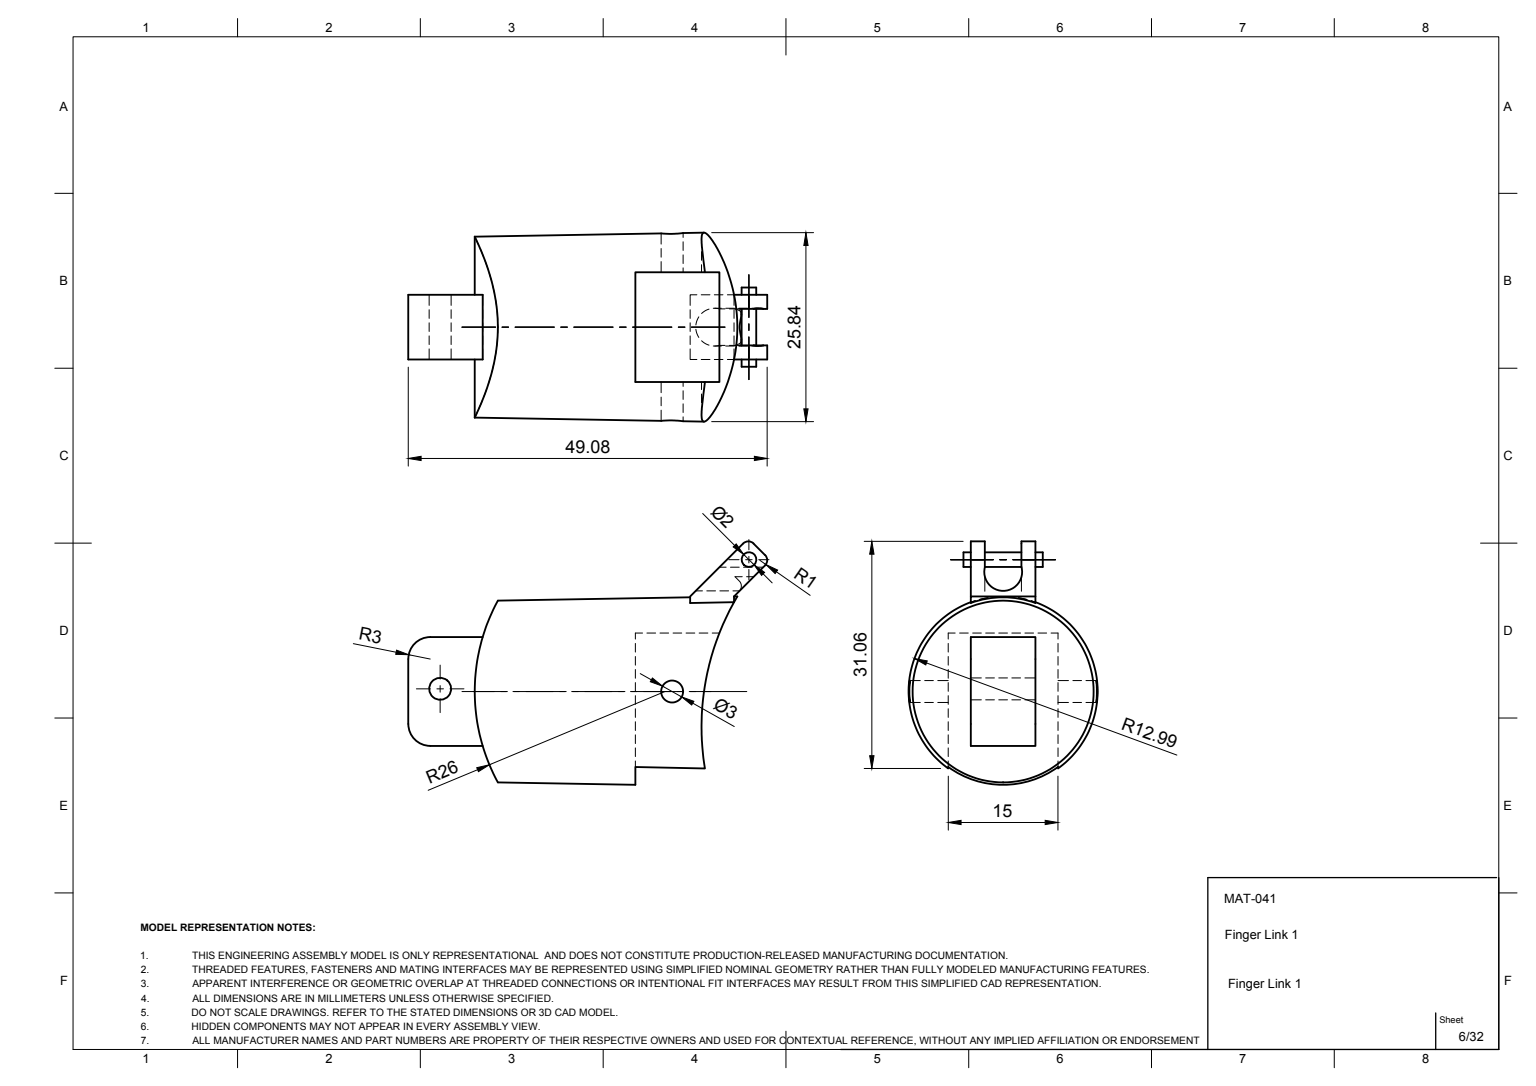
ISO-10303-21;
HEADER;
/* Generated by software containing ST-Developer
 * from STEP Tools, Inc. (www.steptools.com) 
 */

FILE_DESCRIPTION(
/* description */ ('STEP AP214'),
/* implementation_level */ '2;1');

FILE_NAME(
/* name */ 'Finger Link 1.step',
/* time_stamp */ '2026-11-14T21:57:47-08:00',
/* author */ (''),
/* organization */ (''),
/* preprocessor_version */ 'ST-DEVELOPER v20.2',
/* originating_system */ 'Autodesk Translation Framework v15.17.0.0',
/* authorisation */ '');

FILE_SCHEMA (('AUTOMOTIVE_DESIGN { 1 0 10303 214 3 1 1 }'));
ENDSEC;

DATA;
#10=MECHANICAL_DESIGN_GEOMETRIC_PRESENTATION_REPRESENTATION('',(#249),#13199);
#117=CONICAL_SURFACE('',#7216,13.,0.0174532925199433);
#118=CONICAL_SURFACE('',#7226,13.,0.0174532925199433);
#127=B_SPLINE_CURVE_WITH_KNOTS('',3,(#10160,#10161,#10162,#10163,#10164,
#10165,#10166,#10167,#10168,#10169,#10170,#10171,#10172,#10173,#10174,#10175,
#10176,#10177),.UNSPECIFIED.,.F.,.F.,(4,2,2,2,2,2,2,2,4),(-0.625948273254299,
-0.595286193065165,-0.532168206431192,-0.441842646589546,-0.3515170867479,
-0.261191526906255,-0.170865967064609,-0.107747980430636,-0.0770859002412175),
 .UNSPECIFIED.);
#128=B_SPLINE_CURVE_WITH_KNOTS('',3,(#10225,#10226,#10227,#10228,#10229,
#10230,#10231,#10232,#10233,#10234,#10235,#10236,#10237,#10238,#10239,#10240,
#10241,#10242),.UNSPECIFIED.,.F.,.F.,(4,2,2,2,2,2,2,2,4),(1.130849455016,
1.18732607982086,1.24380270462571,1.30024878607951,1.35669486753331,1.41336679321831,
1.4700387189033,1.52669509758432,1.58335147626535),.UNSPECIFIED.);
#129=B_SPLINE_CURVE_WITH_KNOTS('',3,(#10243,#10244,#10245,#10246,#10247,
#10248,#10249,#10250,#10251,#10252,#10253,#10254,#10255,#10256,#10257,#10258,
#10259,#10260,#10261),.UNSPECIFIED.,.F.,.F.,(4,2,2,2,3,2,2,2,4),(0.678347433766657,
0.735003812447681,0.791660191128705,0.848332116813698,0.905004042498691,
0.961450123952495,1.0178962054063,1.07437283021115,1.130849455016),
 .UNSPECIFIED.);
#130=B_SPLINE_CURVE_WITH_KNOTS('',3,(#10265,#10266,#10267,#10268,#10269,
#10270,#10271,#10272,#10273,#10274,#10275,#10276,#10277,#10278,#10279,#10280,
#10281,#10282),.UNSPECIFIED.,.F.,.F.,(4,2,2,2,2,2,2,2,4),(-0.678347433766657,
-0.621691055085633,-0.565034676404609,-0.508362750719616,-0.451690825034623,
-0.39524474358082,-0.338798662127016,-0.282322037322164,-0.225845412517312),
 .UNSPECIFIED.);
#131=B_SPLINE_CURVE_WITH_KNOTS('',3,(#10286,#10287,#10288,#10289,#10290,
#10291,#10292,#10293,#10294,#10295,#10296,#10297,#10298,#10299,#10300,#10301,
#10302,#10303,#10304),.UNSPECIFIED.,.F.,.F.,(4,2,2,2,3,2,2,2,4),(-0.225845412517312,
-0.169368787712459,-0.112892162907607,-0.0564460814538034,0.,0.0566719256849931,
0.113343851369986,0.17000023005101,0.226656608732034),.UNSPECIFIED.);
#132=B_SPLINE_CURVE_WITH_KNOTS('',3,(#10310,#10311,#10312,#10313),
 .UNSPECIFIED.,.F.,.F.,(4,4),(0.0270217399274549,0.0365389400069035),
 .UNSPECIFIED.);
#133=B_SPLINE_CURVE_WITH_KNOTS('',3,(#10315,#10316,#10317,#10318,#10319,
#10320,#10321,#10322,#10323,#10324,#10325,#10326,#10327,#10328,#10329,#10330,
#10331,#10332),.UNSPECIFIED.,.F.,.F.,(4,2,2,2,2,2,2,2,4),(4.40493642535816,
4.46219553041876,4.95875793037621,5.46800962865692,5.97726132693763,6.22066748237464,
6.46407363781164,6.95088594868566,7.16462957817159),.UNSPECIFIED.);
#134=B_SPLINE_CURVE_WITH_KNOTS('',3,(#10334,#10335,#10336,#10337,#10338,
#10339,#10340),.UNSPECIFIED.,.F.,.F.,(4,3,4),(0.0223867113798144,0.0254340142714909,
0.0283877461116507),.UNSPECIFIED.);
#135=B_SPLINE_CURVE_WITH_KNOTS('',3,(#10346,#10347,#10348,#10349,#10350,
#10351,#10352,#10353,#10354,#10355,#10356,#10357,#10358,#10359,#10360,#10361,
#10362,#10363,#10364,#10365,#10366,#10367,#10368,#10369,#10370,#10371),
 .UNSPECIFIED.,.F.,.F.,(4,2,2,2,2,2,2,2,2,2,2,2,4),(3.80610647446318,4.04439914990187,
4.28269182534056,4.75927717621793,5.2342149273987,5.47168380298909,5.70915267857947,
5.94662421983221,6.18409576108494,6.65903884359041,7.13562589625839,7.37391942259238,
7.61221294892637),.UNSPECIFIED.);
#136=B_SPLINE_CURVE_WITH_KNOTS('',3,(#10372,#10373,#10374,#10375,#10376,
#10377,#10378,#10379,#10380,#10381,#10382,#10383,#10384,#10385,#10386,#10387,
#10388,#10389,#10390,#10391,#10392,#10393,#10394,#10395,#10396,#10397),
 .UNSPECIFIED.,.F.,.F.,(4,2,2,2,2,2,2,2,2,2,2,2,4),(0.,0.238293526333989,
0.476587052667979,0.953174105335958,1.42811718784143,1.66558872909416,1.90306027034689,
2.14052914593728,2.37799802152767,2.85293577270844,3.32952112358581,3.5678137990245,
3.80610647446318),.UNSPECIFIED.);
#137=B_SPLINE_CURVE_WITH_KNOTS('',3,(#10401,#10402,#10403,#10404,#10405,
#10406,#10407),.UNSPECIFIED.,.F.,.F.,(4,3,4),(0.0224802824352469,0.0254340142749992,
0.0284813171662554),.UNSPECIFIED.);
#138=B_SPLINE_CURVE_WITH_KNOTS('',3,(#10409,#10410,#10411,#10412,#10413,
#10414,#10415,#10416,#10417,#10418,#10419,#10420,#10421,#10422,#10423,#10424,
#10425,#10426),.UNSPECIFIED.,.F.,.F.,(4,2,2,2,2,2,2,2,4),(0.766636682751041,
0.98038031223697,1.46719262311099,1.710598778548,1.95400493398501,2.46325663226571,
2.97250833054642,3.46907073050387,3.52632983556447),.UNSPECIFIED.);
#139=B_SPLINE_CURVE_WITH_KNOTS('',3,(#10427,#10428,#10429,#10430),
 .UNSPECIFIED.,.F.,.F.,(4,4),(0.0143722070064857,0.0238894070520057),
 .UNSPECIFIED.);
#140=B_SPLINE_CURVE_WITH_KNOTS('',3,(#10456,#10457,#10458,#10459,#10460,
#10461,#10462,#10463,#10464,#10465),.UNSPECIFIED.,.F.,.F.,(4,2,2,2,4),(3.52632983556447,
3.71735193048259,3.96563313046132,4.21391433044004,4.40493642535816),
 .UNSPECIFIED.);
#213=SHAPE_REPRESENTATION_RELATIONSHIP('SRR','None',#13281,#231);
#231=ADVANCED_BREP_SHAPE_REPRESENTATION('',(#267),#13177);
#249=STYLED_ITEM('',(#13409),#267);
#267=MANIFOLD_SOLID_BREP('Body1',#6844);
#290=FACE_BOUND('',#2265,.T.);
#291=FACE_BOUND('',#2266,.T.);
#292=FACE_BOUND('',#2274,.T.);
#293=FACE_BOUND('',#2277,.T.);
#294=FACE_BOUND('',#2279,.T.);
#295=FACE_BOUND('',#2283,.T.);
#296=FACE_BOUND('',#2286,.T.);
#297=FACE_BOUND('',#2292,.T.);
#298=FACE_BOUND('',#2294,.T.);
#299=FACE_BOUND('',#2304,.T.);
#300=FACE_BOUND('',#2307,.T.);
#387=ELLIPSE('',#7195,3.65324790347504,2.58323636587766);
#388=ELLIPSE('',#7196,3.65324790353112,2.58323636594297);
#389=ELLIPSE('',#7197,3.65324790353033,2.58323636594184);
#390=ELLIPSE('',#7198,3.65324790353218,2.58323636594453);
#391=ELLIPSE('',#7199,3.65324790349574,2.58323636589973);
#416=PLANE('',#7220);
#417=PLANE('',#7221);
#418=PLANE('',#7223);
#419=PLANE('',#7225);
#420=PLANE('',#7234);
#421=PLANE('',#7235);
#422=PLANE('',#7236);
#423=PLANE('',#7237);
#424=PLANE('',#7238);
#425=PLANE('',#7239);
#426=PLANE('',#7242);
#427=PLANE('',#7243);
#428=PLANE('',#7246);
#429=PLANE('',#7247);
#430=PLANE('',#7248);
#431=PLANE('',#7249);
#432=PLANE('',#7250);
#433=PLANE('',#7253);
#434=PLANE('',#7256);
#435=PLANE('',#7257);
#436=PLANE('',#7263);
#437=PLANE('',#7264);
#438=PLANE('',#7267);
#439=PLANE('',#7268);
#440=PLANE('',#7271);
#672=LINE('',#10181,#1190);
#673=LINE('',#10185,#1191);
#674=LINE('',#10189,#1192);
#675=LINE('',#10193,#1193);
#676=LINE('',#10199,#1194);
#677=LINE('',#10205,#1195);
#678=LINE('',#10211,#1196);
#679=LINE('',#10217,#1197);
#680=LINE('',#10223,#1198);
#681=LINE('',#10284,#1199);
#682=LINE('',#10344,#1200);
#683=LINE('',#10433,#1201);
#684=LINE('',#10434,#1202);
#685=LINE('',#10437,#1203);
#686=LINE('',#10441,#1204);
#687=LINE('',#10443,#1205);
#688=LINE('',#10448,#1206);
#689=LINE('',#10450,#1207);
#690=LINE('',#10452,#1208);
#691=LINE('',#10453,#1209);
#692=LINE('',#10469,#1210);
#693=LINE('',#10475,#1211);
#694=LINE('',#10479,#1212);
#695=LINE('',#10483,#1213);
#696=LINE('',#10485,#1214);
#697=LINE('',#10486,#1215);
#698=LINE('',#10488,#1216);
#699=LINE('',#10490,#1217);
#700=LINE('',#10494,#1218);
#701=LINE('',#10496,#1219);
#702=LINE('',#10497,#1220);
#703=LINE('',#10501,#1221);
#704=LINE('',#10505,#1222);
#705=LINE('',#10506,#1223);
#706=LINE('',#10508,#1224);
#707=LINE('',#10512,#1225);
#708=LINE('',#10513,#1226);
#709=LINE('',#10516,#1227);
#710=LINE('',#10520,#1228);
#711=LINE('',#10523,#1229);
#712=LINE('',#10524,#1230);
#713=LINE('',#10526,#1231);
#714=LINE('',#10527,#1232);
#715=LINE('',#10528,#1233);
#716=LINE('',#10531,#1234);
#717=LINE('',#10533,#1235);
#718=LINE('',#10534,#1236);
#719=LINE('',#10535,#1237);
#720=LINE('',#10539,#1238);
#721=LINE('',#10540,#1239);
#722=LINE('',#10541,#1240);
#723=LINE('',#10543,#1241);
#724=LINE('',#10560,#1242);
#725=LINE('',#10562,#1243);
#726=LINE('',#10564,#1244);
#727=LINE('',#10565,#1245);
#728=LINE('',#10568,#1246);
#729=LINE('',#10572,#1247);
#730=LINE('',#10575,#1248);
#731=LINE('',#10576,#1249);
#732=LINE('',#10580,#1250);
#733=LINE('',#10583,#1251);
#1190=VECTOR('',#8163,1000.);
#1191=VECTOR('',#8166,1000.);
#1192=VECTOR('',#8169,1000.);
#1193=VECTOR('',#8172,1000.);
#1194=VECTOR('',#8179,1.5);
#1195=VECTOR('',#8186,1.);
#1196=VECTOR('',#8193,1.);
#1197=VECTOR('',#8200,1.);
#1198=VECTOR('',#8207,1.5);
#1199=VECTOR('',#8210,1.5);
#1200=VECTOR('',#8219,13.);
#1201=VECTOR('',#8224,1000.);
#1202=VECTOR('',#8225,1000.);
#1203=VECTOR('',#8228,1000.);
#1204=VECTOR('',#8233,1000.);
#1205=VECTOR('',#8234,1000.);
#1206=VECTOR('',#8239,1000.);
#1207=VECTOR('',#8240,1000.);
#1208=VECTOR('',#8241,1000.);
#1209=VECTOR('',#8242,1000.);
#1210=VECTOR('',#8249,1000.);
#1211=VECTOR('',#8256,1000.);
#1212=VECTOR('',#8259,1000.);
#1213=VECTOR('',#8264,1000.);
#1214=VECTOR('',#8265,1000.);
#1215=VECTOR('',#8266,1000.);
#1216=VECTOR('',#8269,1000.);
#1217=VECTOR('',#8272,1000.);
#1218=VECTOR('',#8277,1000.);
#1219=VECTOR('',#8278,1000.);
#1220=VECTOR('',#8279,1000.);
#1221=VECTOR('',#8282,1000.);
#1222=VECTOR('',#8285,1000.);
#1223=VECTOR('',#8286,1000.);
#1224=VECTOR('',#8287,1000.);
#1225=VECTOR('',#8292,1000.);
#1226=VECTOR('',#8293,1000.);
#1227=VECTOR('',#8296,1000.);
#1228=VECTOR('',#8301,1000.);
#1229=VECTOR('',#8304,1000.);
#1230=VECTOR('',#8305,1000.);
#1231=VECTOR('',#8306,1000.);
#1232=VECTOR('',#8307,1000.);
#1233=VECTOR('',#8308,1000.);
#1234=VECTOR('',#8311,1000.);
#1235=VECTOR('',#8312,1000.);
#1236=VECTOR('',#8313,1000.);
#1237=VECTOR('',#8314,1000.);
#1238=VECTOR('',#8317,1000.);
#1239=VECTOR('',#8318,1000.);
#1240=VECTOR('',#8319,1000.);
#1241=VECTOR('',#8322,1000.);
#1242=VECTOR('',#8351,1000.);
#1243=VECTOR('',#8352,1000.);
#1244=VECTOR('',#8353,1000.);
#1245=VECTOR('',#8354,1000.);
#1246=VECTOR('',#8357,1000.);
#1247=VECTOR('',#8362,1000.);
#1248=VECTOR('',#8365,1000.);
#1249=VECTOR('',#8366,1000.);
#1250=VECTOR('',#8371,1000.);
#1251=VECTOR('',#8376,1000.);
#1669=CYLINDRICAL_SURFACE('',#7194,2.58323636594183);
#1670=CYLINDRICAL_SURFACE('',#7200,1.5);
#1671=CYLINDRICAL_SURFACE('',#7203,1.);
#1672=CYLINDRICAL_SURFACE('',#7206,1.);
#1673=CYLINDRICAL_SURFACE('',#7209,1.);
#1674=CYLINDRICAL_SURFACE('',#7212,1.5);
#1675=CYLINDRICAL_SURFACE('',#7214,1.5);
#1676=CYLINDRICAL_SURFACE('',#7228,35.);
#1677=CYLINDRICAL_SURFACE('',#7231,26.);
#1678=CYLINDRICAL_SURFACE('',#7258,1.);
#1679=CYLINDRICAL_SURFACE('',#7259,1.);
#1680=CYLINDRICAL_SURFACE('',#7260,1.);
#1681=CYLINDRICAL_SURFACE('',#7261,1.);
#1682=CYLINDRICAL_SURFACE('',#7262,1.);
#1683=CYLINDRICAL_SURFACE('',#7272,3.);
#1684=CYLINDRICAL_SURFACE('',#7273,3.);
#1860=FACE_OUTER_BOUND('',#2257,.T.);
#1861=FACE_OUTER_BOUND('',#2258,.T.);
#1862=FACE_OUTER_BOUND('',#2259,.T.);
#1863=FACE_OUTER_BOUND('',#2260,.T.);
#1864=FACE_OUTER_BOUND('',#2261,.T.);
#1865=FACE_OUTER_BOUND('',#2262,.T.);
#1866=FACE_OUTER_BOUND('',#2263,.T.);
#1867=FACE_OUTER_BOUND('',#2264,.T.);
#1868=FACE_OUTER_BOUND('',#2267,.T.);
#1869=FACE_OUTER_BOUND('',#2268,.T.);
#1870=FACE_OUTER_BOUND('',#2269,.T.);
#1871=FACE_OUTER_BOUND('',#2270,.T.);
#1872=FACE_OUTER_BOUND('',#2271,.T.);
#1873=FACE_OUTER_BOUND('',#2272,.T.);
#1874=FACE_OUTER_BOUND('',#2273,.T.);
#1875=FACE_OUTER_BOUND('',#2275,.T.);
#1876=FACE_OUTER_BOUND('',#2276,.T.);
#1877=FACE_OUTER_BOUND('',#2278,.T.);
#1878=FACE_OUTER_BOUND('',#2280,.T.);
#1879=FACE_OUTER_BOUND('',#2281,.T.);
#1880=FACE_OUTER_BOUND('',#2282,.T.);
#1881=FACE_OUTER_BOUND('',#2284,.T.);
#1882=FACE_OUTER_BOUND('',#2285,.T.);
#1883=FACE_OUTER_BOUND('',#2287,.T.);
#1884=FACE_OUTER_BOUND('',#2288,.T.);
#1885=FACE_OUTER_BOUND('',#2289,.T.);
#1886=FACE_OUTER_BOUND('',#2290,.T.);
#1887=FACE_OUTER_BOUND('',#2291,.T.);
#1888=FACE_OUTER_BOUND('',#2293,.T.);
#1889=FACE_OUTER_BOUND('',#2295,.T.);
#1890=FACE_OUTER_BOUND('',#2296,.T.);
#1891=FACE_OUTER_BOUND('',#2297,.T.);
#1892=FACE_OUTER_BOUND('',#2298,.T.);
#1893=FACE_OUTER_BOUND('',#2299,.T.);
#1894=FACE_OUTER_BOUND('',#2300,.T.);
#1895=FACE_OUTER_BOUND('',#2301,.T.);
#1896=FACE_OUTER_BOUND('',#2302,.T.);
#1897=FACE_OUTER_BOUND('',#2303,.T.);
#1898=FACE_OUTER_BOUND('',#2305,.T.);
#1899=FACE_OUTER_BOUND('',#2306,.T.);
#1900=FACE_OUTER_BOUND('',#2308,.T.);
#1901=FACE_OUTER_BOUND('',#2309,.T.);
#1902=FACE_OUTER_BOUND('',#2310,.T.);
#2257=EDGE_LOOP('',(#4822,#4823,#4824,#4825,#4826,#4827,#4828,#4829,#4830,
#4831));
#2258=EDGE_LOOP('',(#4832,#4833,#4834,#4835));
#2259=EDGE_LOOP('',(#4836,#4837,#4838,#4839));
#2260=EDGE_LOOP('',(#4840,#4841,#4842,#4843));
#2261=EDGE_LOOP('',(#4844,#4845,#4846,#4847));
#2262=EDGE_LOOP('',(#4848,#4849,#4850,#4851,#4852));
#2263=EDGE_LOOP('',(#4853,#4854,#4855,#4856,#4857));
#2264=EDGE_LOOP('',(#4858,#4859,#4860,#4861,#4862,#4863,#4864,#4865,#4866,
#4867,#4868,#4869,#4870));
#2265=EDGE_LOOP('',(#4871,#4872));
#2266=EDGE_LOOP('',(#4873,#4874));
#2267=EDGE_LOOP('',(#4875,#4876,#4877));
#2268=EDGE_LOOP('',(#4878,#4879,#4880,#4881));
#2269=EDGE_LOOP('',(#4882,#4883,#4884,#4885));
#2270=EDGE_LOOP('',(#4886,#4887,#4888,#4889));
#2271=EDGE_LOOP('',(#4890,#4891));
#2272=EDGE_LOOP('',(#4892,#4893,#4894,#4895,#4896,#4897));
#2273=EDGE_LOOP('',(#4898,#4899));
#2274=EDGE_LOOP('',(#4900,#4901,#4902,#4903));
#2275=EDGE_LOOP('',(#4904,#4905,#4906,#4907));
#2276=EDGE_LOOP('',(#4908,#4909,#4910,#4911));
#2277=EDGE_LOOP('',(#4912));
#2278=EDGE_LOOP('',(#4913,#4914,#4915,#4916));
#2279=EDGE_LOOP('',(#4917));
#2280=EDGE_LOOP('',(#4918,#4919,#4920,#4921));
#2281=EDGE_LOOP('',(#4922,#4923,#4924,#4925));
#2282=EDGE_LOOP('',(#4926,#4927,#4928,#4929,#4930,#4931,#4932,#4933));
#2283=EDGE_LOOP('',(#4934));
#2284=EDGE_LOOP('',(#4935,#4936,#4937,#4938,#4939));
#2285=EDGE_LOOP('',(#4940,#4941,#4942,#4943,#4944,#4945,#4946,#4947));
#2286=EDGE_LOOP('',(#4948));
#2287=EDGE_LOOP('',(#4949,#4950,#4951,#4952,#4953,#4954,#4955,#4956,#4957,
#4958,#4959,#4960));
#2288=EDGE_LOOP('',(#4961,#4962,#4963,#4964,#4965,#4966,#4967,#4968));
#2289=EDGE_LOOP('',(#4969,#4970,#4971,#4972));
#2290=EDGE_LOOP('',(#4973,#4974,#4975));
#2291=EDGE_LOOP('',(#4976,#4977,#4978,#4979,#4980,#4981));
#2292=EDGE_LOOP('',(#4982));
#2293=EDGE_LOOP('',(#4983,#4984,#4985,#4986,#4987,#4988));
#2294=EDGE_LOOP('',(#4989));
#2295=EDGE_LOOP('',(#4990));
#2296=EDGE_LOOP('',(#4991));
#2297=EDGE_LOOP('',(#4992,#4993,#4994,#4995));
#2298=EDGE_LOOP('',(#4996,#4997,#4998,#4999));
#2299=EDGE_LOOP('',(#5000,#5001,#5002,#5003));
#2300=EDGE_LOOP('',(#5004,#5005,#5006,#5007));
#2301=EDGE_LOOP('',(#5008,#5009,#5010,#5011,#5012,#5013));
#2302=EDGE_LOOP('',(#5014,#5015,#5016,#5017));
#2303=EDGE_LOOP('',(#5018,#5019,#5020,#5021,#5022,#5023));
#2304=EDGE_LOOP('',(#5024));
#2305=EDGE_LOOP('',(#5025,#5026,#5027,#5028));
#2306=EDGE_LOOP('',(#5029,#5030,#5031,#5032,#5033,#5034));
#2307=EDGE_LOOP('',(#5035));
#2308=EDGE_LOOP('',(#5036,#5037,#5038,#5039));
#2309=EDGE_LOOP('',(#5040,#5041,#5042,#5043));
#2310=EDGE_LOOP('',(#5044,#5045,#5046,#5047));
#2747=CIRCLE('',#7201,1.5);
#2748=CIRCLE('',#7202,1.5);
#2749=CIRCLE('',#7204,1.);
#2750=CIRCLE('',#7205,1.);
#2751=CIRCLE('',#7207,1.);
#2752=CIRCLE('',#7208,1.);
#2753=CIRCLE('',#7210,1.);
#2754=CIRCLE('',#7211,1.);
#2755=CIRCLE('',#7213,1.5);
#2756=CIRCLE('',#7215,1.5);
#2757=CIRCLE('',#7217,12.7565008166693);
#2758=CIRCLE('',#7218,12.8874008156035);
#2759=CIRCLE('',#7219,12.8874008156035);
#2760=CIRCLE('',#7222,1.);
#2761=CIRCLE('',#7224,1.);
#2762=CIRCLE('',#7227,12.9921312051728);
#2763=CIRCLE('',#7229,35.);
#2764=CIRCLE('',#7230,35.);
#2765=CIRCLE('',#7232,26.);
#2766=CIRCLE('',#7233,26.);
#2767=CIRCLE('',#7240,1.);
#2768=CIRCLE('',#7241,1.);
#2769=CIRCLE('',#7244,1.);
#2770=CIRCLE('',#7245,1.);
#2771=CIRCLE('',#7251,1.);
#2772=CIRCLE('',#7252,1.);
#2773=CIRCLE('',#7254,1.);
#2774=CIRCLE('',#7255,1.);
#2775=CIRCLE('',#7265,3.);
#2776=CIRCLE('',#7266,3.);
#2777=CIRCLE('',#7269,3.);
#2778=CIRCLE('',#7270,3.);
#3076=VERTEX_POINT('',#10158);
#3077=VERTEX_POINT('',#10159);
#3078=VERTEX_POINT('',#10178);
#3079=VERTEX_POINT('',#10180);
#3080=VERTEX_POINT('',#10182);
#3081=VERTEX_POINT('',#10184);
#3082=VERTEX_POINT('',#10186);
#3083=VERTEX_POINT('',#10188);
#3084=VERTEX_POINT('',#10190);
#3085=VERTEX_POINT('',#10192);
#3086=VERTEX_POINT('',#10196);
#3087=VERTEX_POINT('',#10198);
#3088=VERTEX_POINT('',#10202);
#3089=VERTEX_POINT('',#10204);
#3090=VERTEX_POINT('',#10208);
#3091=VERTEX_POINT('',#10210);
#3092=VERTEX_POINT('',#10214);
#3093=VERTEX_POINT('',#10216);
#3094=VERTEX_POINT('',#10220);
#3095=VERTEX_POINT('',#10222);
#3096=VERTEX_POINT('',#10224);
#3097=VERTEX_POINT('',#10263);
#3098=VERTEX_POINT('',#10264);
#3099=VERTEX_POINT('',#10283);
#3100=VERTEX_POINT('',#10306);
#3101=VERTEX_POINT('',#10307);
#3102=VERTEX_POINT('',#10309);
#3103=VERTEX_POINT('',#10314);
#3104=VERTEX_POINT('',#10333);
#3105=VERTEX_POINT('',#10341);
#3106=VERTEX_POINT('',#10343);
#3107=VERTEX_POINT('',#10345);
#3108=VERTEX_POINT('',#10398);
#3109=VERTEX_POINT('',#10400);
#3110=VERTEX_POINT('',#10408);
#3111=VERTEX_POINT('',#10432);
#3112=VERTEX_POINT('',#10436);
#3113=VERTEX_POINT('',#10440);
#3114=VERTEX_POINT('',#10442);
#3115=VERTEX_POINT('',#10446);
#3116=VERTEX_POINT('',#10447);
#3117=VERTEX_POINT('',#10449);
#3118=VERTEX_POINT('',#10451);
#3119=VERTEX_POINT('',#10467);
#3120=VERTEX_POINT('',#10468);
#3121=VERTEX_POINT('',#10473);
#3122=VERTEX_POINT('',#10474);
#3123=VERTEX_POINT('',#10476);
#3124=VERTEX_POINT('',#10478);
#3125=VERTEX_POINT('',#10482);
#3126=VERTEX_POINT('',#10484);
#3127=VERTEX_POINT('',#10493);
#3128=VERTEX_POINT('',#10495);
#3129=VERTEX_POINT('',#10499);
#3130=VERTEX_POINT('',#10500);
#3131=VERTEX_POINT('',#10502);
#3132=VERTEX_POINT('',#10504);
#3133=VERTEX_POINT('',#10507);
#3134=VERTEX_POINT('',#10511);
#3135=VERTEX_POINT('',#10515);
#3136=VERTEX_POINT('',#10518);
#3137=VERTEX_POINT('',#10522);
#3138=VERTEX_POINT('',#10525);
#3139=VERTEX_POINT('',#10530);
#3140=VERTEX_POINT('',#10532);
#3141=VERTEX_POINT('',#10537);
#3142=VERTEX_POINT('',#10538);
#3143=VERTEX_POINT('',#10558);
#3144=VERTEX_POINT('',#10559);
#3145=VERTEX_POINT('',#10561);
#3146=VERTEX_POINT('',#10563);
#3147=VERTEX_POINT('',#10567);
#3148=VERTEX_POINT('',#10570);
#3149=VERTEX_POINT('',#10574);
#3150=VERTEX_POINT('',#10579);
#3748=EDGE_CURVE('',#3076,#3077,#127,.T.);
#3749=EDGE_CURVE('',#3078,#3077,#387,.T.);
#3750=EDGE_CURVE('',#3079,#3078,#672,.T.);
#3751=EDGE_CURVE('',#3080,#3079,#388,.T.);
#3752=EDGE_CURVE('',#3080,#3081,#673,.T.);
#3753=EDGE_CURVE('',#3082,#3081,#389,.T.);
#3754=EDGE_CURVE('',#3083,#3082,#674,.T.);
#3755=EDGE_CURVE('',#3084,#3083,#390,.T.);
#3756=EDGE_CURVE('',#3085,#3084,#675,.T.);
#3757=EDGE_CURVE('',#3076,#3085,#391,.T.);
#3758=EDGE_CURVE('',#3086,#3086,#2747,.T.);
#3759=EDGE_CURVE('',#3086,#3087,#676,.T.);
#3760=EDGE_CURVE('',#3087,#3087,#2748,.T.);
#3761=EDGE_CURVE('',#3088,#3088,#2749,.T.);
#3762=EDGE_CURVE('',#3088,#3089,#677,.T.);
#3763=EDGE_CURVE('',#3089,#3089,#2750,.T.);
#3764=EDGE_CURVE('',#3090,#3090,#2751,.T.);
#3765=EDGE_CURVE('',#3090,#3091,#678,.T.);
#3766=EDGE_CURVE('',#3091,#3091,#2752,.T.);
#3767=EDGE_CURVE('',#3092,#3092,#2753,.T.);
#3768=EDGE_CURVE('',#3092,#3093,#679,.T.);
#3769=EDGE_CURVE('',#3093,#3093,#2754,.T.);
#3770=EDGE_CURVE('',#3094,#3094,#2755,.T.);
#3771=EDGE_CURVE('',#3094,#3095,#680,.T.);
#3772=EDGE_CURVE('',#3095,#3096,#128,.T.);
#3773=EDGE_CURVE('',#3096,#3095,#129,.T.);
#3774=EDGE_CURVE('',#3097,#3098,#130,.T.);
#3775=EDGE_CURVE('',#3098,#3099,#681,.T.);
#3776=EDGE_CURVE('',#3099,#3099,#2756,.T.);
#3777=EDGE_CURVE('',#3098,#3097,#131,.T.);
#3778=EDGE_CURVE('',#3100,#3101,#2757,.T.);
#3779=EDGE_CURVE('',#3102,#3100,#132,.T.);
#3780=EDGE_CURVE('',#3103,#3102,#133,.T.);
#3781=EDGE_CURVE('',#3103,#3104,#134,.T.);
#3782=EDGE_CURVE('',#3104,#3105,#2758,.T.);
#3783=EDGE_CURVE('',#3105,#3106,#682,.T.);
#3784=EDGE_CURVE('',#3106,#3107,#135,.T.);
#3785=EDGE_CURVE('',#3107,#3106,#136,.T.);
#3786=EDGE_CURVE('',#3105,#3108,#2759,.T.);
#3787=EDGE_CURVE('',#3108,#3109,#137,.T.);
#3788=EDGE_CURVE('',#3110,#3109,#138,.T.);
#3789=EDGE_CURVE('',#3101,#3110,#139,.T.);
#3790=EDGE_CURVE('',#3111,#3078,#683,.T.);
#3791=EDGE_CURVE('',#3077,#3111,#684,.T.);
#3792=EDGE_CURVE('',#3079,#3112,#685,.T.);
#3793=EDGE_CURVE('',#3111,#3112,#2760,.T.);
#3794=EDGE_CURVE('',#3113,#3085,#686,.T.);
#3795=EDGE_CURVE('',#3114,#3084,#687,.T.);
#3796=EDGE_CURVE('',#3114,#3113,#2761,.T.);
#3797=EDGE_CURVE('',#3115,#3116,#688,.T.);
#3798=EDGE_CURVE('',#3116,#3117,#689,.T.);
#3799=EDGE_CURVE('',#3118,#3117,#690,.T.);
#3800=EDGE_CURVE('',#3118,#3115,#691,.T.);
#3801=EDGE_CURVE('',#3109,#3103,#2762,.T.);
#3802=EDGE_CURVE('',#3109,#3103,#140,.T.);
#3803=EDGE_CURVE('',#3119,#3120,#692,.T.);
#3804=EDGE_CURVE('',#3119,#3110,#2763,.T.);
#3805=EDGE_CURVE('',#3102,#3120,#2764,.T.);
#3806=EDGE_CURVE('',#3121,#3122,#693,.T.);
#3807=EDGE_CURVE('',#3123,#3121,#2765,.T.);
#3808=EDGE_CURVE('',#3124,#3123,#694,.T.);
#3809=EDGE_CURVE('',#3122,#3124,#2766,.T.);
#3810=EDGE_CURVE('',#3101,#3125,#695,.T.);
#3811=EDGE_CURVE('',#3126,#3125,#696,.T.);
#3812=EDGE_CURVE('',#3100,#3126,#697,.T.);
#3813=EDGE_CURVE('',#3125,#3119,#698,.T.);
#3814=EDGE_CURVE('',#3120,#3126,#699,.T.);
#3815=EDGE_CURVE('',#3109,#3127,#700,.T.);
#3816=EDGE_CURVE('',#3127,#3128,#701,.T.);
#3817=EDGE_CURVE('',#3103,#3128,#702,.T.);
#3818=EDGE_CURVE('',#3129,#3130,#703,.T.);
#3819=EDGE_CURVE('',#3129,#3131,#2767,.T.);
#3820=EDGE_CURVE('',#3131,#3132,#704,.T.);
#3821=EDGE_CURVE('',#3104,#3132,#705,.T.);
#3822=EDGE_CURVE('',#3133,#3128,#706,.T.);
#3823=EDGE_CURVE('',#3133,#3130,#2768,.T.);
#3824=EDGE_CURVE('',#3132,#3134,#707,.T.);
#3825=EDGE_CURVE('',#3108,#3134,#708,.T.);
#3826=EDGE_CURVE('',#3135,#3134,#709,.T.);
#3827=EDGE_CURVE('',#3135,#3116,#2769,.T.);
#3828=EDGE_CURVE('',#3115,#3136,#2770,.T.);
#3829=EDGE_CURVE('',#3136,#3127,#710,.T.);
#3830=EDGE_CURVE('',#3083,#3137,#711,.T.);
#3831=EDGE_CURVE('',#3137,#3133,#712,.T.);
#3832=EDGE_CURVE('',#3136,#3138,#713,.T.);
#3833=EDGE_CURVE('',#3138,#3080,#714,.T.);
#3834=EDGE_CURVE('',#3112,#3114,#715,.T.);
#3835=EDGE_CURVE('',#3082,#3139,#716,.T.);
#3836=EDGE_CURVE('',#3140,#3081,#717,.T.);
#3837=EDGE_CURVE('',#3140,#3135,#718,.T.);
#3838=EDGE_CURVE('',#3131,#3139,#719,.T.);
#3839=EDGE_CURVE('',#3141,#3142,#720,.T.);
#3840=EDGE_CURVE('',#3141,#3129,#721,.T.);
#3841=EDGE_CURVE('',#3130,#3142,#722,.T.);
#3842=EDGE_CURVE('',#3113,#3076,#723,.T.);
#3843=EDGE_CURVE('',#3138,#3118,#2771,.T.);
#3844=EDGE_CURVE('',#3117,#3140,#2772,.T.);
#3845=EDGE_CURVE('',#3139,#3141,#2773,.T.);
#3846=EDGE_CURVE('',#3142,#3137,#2774,.T.);
#3847=EDGE_CURVE('',#3143,#3144,#724,.T.);
#3848=EDGE_CURVE('',#3144,#3145,#725,.T.);
#3849=EDGE_CURVE('',#3145,#3146,#726,.T.);
#3850=EDGE_CURVE('',#3146,#3143,#727,.T.);
#3851=EDGE_CURVE('',#3121,#3147,#728,.T.);
#3852=EDGE_CURVE('',#3147,#3144,#2775,.T.);
#3853=EDGE_CURVE('',#3143,#3148,#2776,.T.);
#3854=EDGE_CURVE('',#3123,#3148,#729,.T.);
#3855=EDGE_CURVE('',#3122,#3149,#730,.T.);
#3856=EDGE_CURVE('',#3149,#3147,#731,.T.);
#3857=EDGE_CURVE('',#3145,#3149,#2777,.T.);
#3858=EDGE_CURVE('',#3124,#3150,#732,.T.);
#3859=EDGE_CURVE('',#3150,#3146,#2778,.T.);
#3860=EDGE_CURVE('',#3148,#3150,#733,.T.);
#4822=ORIENTED_EDGE('',*,*,#3748,.T.);
#4823=ORIENTED_EDGE('',*,*,#3749,.F.);
#4824=ORIENTED_EDGE('',*,*,#3750,.F.);
#4825=ORIENTED_EDGE('',*,*,#3751,.F.);
#4826=ORIENTED_EDGE('',*,*,#3752,.T.);
#4827=ORIENTED_EDGE('',*,*,#3753,.F.);
#4828=ORIENTED_EDGE('',*,*,#3754,.F.);
#4829=ORIENTED_EDGE('',*,*,#3755,.F.);
#4830=ORIENTED_EDGE('',*,*,#3756,.F.);
#4831=ORIENTED_EDGE('',*,*,#3757,.F.);
#4832=ORIENTED_EDGE('',*,*,#3758,.T.);
#4833=ORIENTED_EDGE('',*,*,#3759,.T.);
#4834=ORIENTED_EDGE('',*,*,#3760,.T.);
#4835=ORIENTED_EDGE('',*,*,#3759,.F.);
#4836=ORIENTED_EDGE('',*,*,#3761,.T.);
#4837=ORIENTED_EDGE('',*,*,#3762,.T.);
#4838=ORIENTED_EDGE('',*,*,#3763,.T.);
#4839=ORIENTED_EDGE('',*,*,#3762,.F.);
#4840=ORIENTED_EDGE('',*,*,#3764,.T.);
#4841=ORIENTED_EDGE('',*,*,#3765,.T.);
#4842=ORIENTED_EDGE('',*,*,#3766,.F.);
#4843=ORIENTED_EDGE('',*,*,#3765,.F.);
#4844=ORIENTED_EDGE('',*,*,#3767,.T.);
#4845=ORIENTED_EDGE('',*,*,#3768,.T.);
#4846=ORIENTED_EDGE('',*,*,#3769,.T.);
#4847=ORIENTED_EDGE('',*,*,#3768,.F.);
#4848=ORIENTED_EDGE('',*,*,#3770,.F.);
#4849=ORIENTED_EDGE('',*,*,#3771,.T.);
#4850=ORIENTED_EDGE('',*,*,#3772,.T.);
#4851=ORIENTED_EDGE('',*,*,#3773,.T.);
#4852=ORIENTED_EDGE('',*,*,#3771,.F.);
#4853=ORIENTED_EDGE('',*,*,#3774,.T.);
#4854=ORIENTED_EDGE('',*,*,#3775,.T.);
#4855=ORIENTED_EDGE('',*,*,#3776,.F.);
#4856=ORIENTED_EDGE('',*,*,#3775,.F.);
#4857=ORIENTED_EDGE('',*,*,#3777,.T.);
#4858=ORIENTED_EDGE('',*,*,#3778,.F.);
#4859=ORIENTED_EDGE('',*,*,#3779,.F.);
#4860=ORIENTED_EDGE('',*,*,#3780,.F.);
#4861=ORIENTED_EDGE('',*,*,#3781,.T.);
#4862=ORIENTED_EDGE('',*,*,#3782,.T.);
#4863=ORIENTED_EDGE('',*,*,#3783,.T.);
#4864=ORIENTED_EDGE('',*,*,#3784,.T.);
#4865=ORIENTED_EDGE('',*,*,#3785,.T.);
#4866=ORIENTED_EDGE('',*,*,#3783,.F.);
#4867=ORIENTED_EDGE('',*,*,#3786,.T.);
#4868=ORIENTED_EDGE('',*,*,#3787,.T.);
#4869=ORIENTED_EDGE('',*,*,#3788,.F.);
#4870=ORIENTED_EDGE('',*,*,#3789,.F.);
#4871=ORIENTED_EDGE('',*,*,#3774,.F.);
#4872=ORIENTED_EDGE('',*,*,#3777,.F.);
#4873=ORIENTED_EDGE('',*,*,#3773,.F.);
#4874=ORIENTED_EDGE('',*,*,#3772,.F.);
#4875=ORIENTED_EDGE('',*,*,#3790,.T.);
#4876=ORIENTED_EDGE('',*,*,#3749,.T.);
#4877=ORIENTED_EDGE('',*,*,#3791,.T.);
#4878=ORIENTED_EDGE('',*,*,#3792,.F.);
#4879=ORIENTED_EDGE('',*,*,#3750,.T.);
#4880=ORIENTED_EDGE('',*,*,#3790,.F.);
#4881=ORIENTED_EDGE('',*,*,#3793,.T.);
#4882=ORIENTED_EDGE('',*,*,#3794,.T.);
#4883=ORIENTED_EDGE('',*,*,#3756,.T.);
#4884=ORIENTED_EDGE('',*,*,#3795,.F.);
#4885=ORIENTED_EDGE('',*,*,#3796,.T.);
#4886=ORIENTED_EDGE('',*,*,#3797,.T.);
#4887=ORIENTED_EDGE('',*,*,#3798,.T.);
#4888=ORIENTED_EDGE('',*,*,#3799,.F.);
#4889=ORIENTED_EDGE('',*,*,#3800,.T.);
#4890=ORIENTED_EDGE('',*,*,#3801,.T.);
#4891=ORIENTED_EDGE('',*,*,#3802,.F.);
#4892=ORIENTED_EDGE('',*,*,#3803,.F.);
#4893=ORIENTED_EDGE('',*,*,#3804,.T.);
#4894=ORIENTED_EDGE('',*,*,#3788,.T.);
#4895=ORIENTED_EDGE('',*,*,#3802,.T.);
#4896=ORIENTED_EDGE('',*,*,#3780,.T.);
#4897=ORIENTED_EDGE('',*,*,#3805,.T.);
#4898=ORIENTED_EDGE('',*,*,#3785,.F.);
#4899=ORIENTED_EDGE('',*,*,#3784,.F.);
#4900=ORIENTED_EDGE('',*,*,#3806,.F.);
#4901=ORIENTED_EDGE('',*,*,#3807,.F.);
#4902=ORIENTED_EDGE('',*,*,#3808,.F.);
#4903=ORIENTED_EDGE('',*,*,#3809,.F.);
#4904=ORIENTED_EDGE('',*,*,#3778,.T.);
#4905=ORIENTED_EDGE('',*,*,#3810,.T.);
#4906=ORIENTED_EDGE('',*,*,#3811,.F.);
#4907=ORIENTED_EDGE('',*,*,#3812,.F.);
#4908=ORIENTED_EDGE('',*,*,#3789,.T.);
#4909=ORIENTED_EDGE('',*,*,#3804,.F.);
#4910=ORIENTED_EDGE('',*,*,#3813,.F.);
#4911=ORIENTED_EDGE('',*,*,#3810,.F.);
#4912=ORIENTED_EDGE('',*,*,#3770,.T.);
#4913=ORIENTED_EDGE('',*,*,#3779,.T.);
#4914=ORIENTED_EDGE('',*,*,#3812,.T.);
#4915=ORIENTED_EDGE('',*,*,#3814,.F.);
#4916=ORIENTED_EDGE('',*,*,#3805,.F.);
#4917=ORIENTED_EDGE('',*,*,#3776,.T.);
#4918=ORIENTED_EDGE('',*,*,#3803,.T.);
#4919=ORIENTED_EDGE('',*,*,#3814,.T.);
#4920=ORIENTED_EDGE('',*,*,#3811,.T.);
#4921=ORIENTED_EDGE('',*,*,#3813,.T.);
#4922=ORIENTED_EDGE('',*,*,#3801,.F.);
#4923=ORIENTED_EDGE('',*,*,#3815,.T.);
#4924=ORIENTED_EDGE('',*,*,#3816,.T.);
#4925=ORIENTED_EDGE('',*,*,#3817,.F.);
#4926=ORIENTED_EDGE('',*,*,#3818,.F.);
#4927=ORIENTED_EDGE('',*,*,#3819,.T.);
#4928=ORIENTED_EDGE('',*,*,#3820,.T.);
#4929=ORIENTED_EDGE('',*,*,#3821,.F.);
#4930=ORIENTED_EDGE('',*,*,#3781,.F.);
#4931=ORIENTED_EDGE('',*,*,#3817,.T.);
#4932=ORIENTED_EDGE('',*,*,#3822,.F.);
#4933=ORIENTED_EDGE('',*,*,#3823,.T.);
#4934=ORIENTED_EDGE('',*,*,#3763,.F.);
#4935=ORIENTED_EDGE('',*,*,#3782,.F.);
#4936=ORIENTED_EDGE('',*,*,#3821,.T.);
#4937=ORIENTED_EDGE('',*,*,#3824,.T.);
#4938=ORIENTED_EDGE('',*,*,#3825,.F.);
#4939=ORIENTED_EDGE('',*,*,#3786,.F.);
#4940=ORIENTED_EDGE('',*,*,#3826,.F.);
#4941=ORIENTED_EDGE('',*,*,#3827,.T.);
#4942=ORIENTED_EDGE('',*,*,#3797,.F.);
#4943=ORIENTED_EDGE('',*,*,#3828,.T.);
#4944=ORIENTED_EDGE('',*,*,#3829,.T.);
#4945=ORIENTED_EDGE('',*,*,#3815,.F.);
#4946=ORIENTED_EDGE('',*,*,#3787,.F.);
#4947=ORIENTED_EDGE('',*,*,#3825,.T.);
#4948=ORIENTED_EDGE('',*,*,#3764,.F.);
#4949=ORIENTED_EDGE('',*,*,#3795,.T.);
#4950=ORIENTED_EDGE('',*,*,#3755,.T.);
#4951=ORIENTED_EDGE('',*,*,#3830,.T.);
#4952=ORIENTED_EDGE('',*,*,#3831,.T.);
#4953=ORIENTED_EDGE('',*,*,#3822,.T.);
#4954=ORIENTED_EDGE('',*,*,#3816,.F.);
#4955=ORIENTED_EDGE('',*,*,#3829,.F.);
#4956=ORIENTED_EDGE('',*,*,#3832,.T.);
#4957=ORIENTED_EDGE('',*,*,#3833,.T.);
#4958=ORIENTED_EDGE('',*,*,#3751,.T.);
#4959=ORIENTED_EDGE('',*,*,#3792,.T.);
#4960=ORIENTED_EDGE('',*,*,#3834,.T.);
#4961=ORIENTED_EDGE('',*,*,#3835,.F.);
#4962=ORIENTED_EDGE('',*,*,#3753,.T.);
#4963=ORIENTED_EDGE('',*,*,#3836,.F.);
#4964=ORIENTED_EDGE('',*,*,#3837,.T.);
#4965=ORIENTED_EDGE('',*,*,#3826,.T.);
#4966=ORIENTED_EDGE('',*,*,#3824,.F.);
#4967=ORIENTED_EDGE('',*,*,#3820,.F.);
#4968=ORIENTED_EDGE('',*,*,#3838,.T.);
#4969=ORIENTED_EDGE('',*,*,#3839,.F.);
#4970=ORIENTED_EDGE('',*,*,#3840,.T.);
#4971=ORIENTED_EDGE('',*,*,#3818,.T.);
#4972=ORIENTED_EDGE('',*,*,#3841,.T.);
#4973=ORIENTED_EDGE('',*,*,#3842,.T.);
#4974=ORIENTED_EDGE('',*,*,#3757,.T.);
#4975=ORIENTED_EDGE('',*,*,#3794,.F.);
#4976=ORIENTED_EDGE('',*,*,#3836,.T.);
#4977=ORIENTED_EDGE('',*,*,#3752,.F.);
#4978=ORIENTED_EDGE('',*,*,#3833,.F.);
#4979=ORIENTED_EDGE('',*,*,#3843,.T.);
#4980=ORIENTED_EDGE('',*,*,#3799,.T.);
#4981=ORIENTED_EDGE('',*,*,#3844,.T.);
#4982=ORIENTED_EDGE('',*,*,#3769,.F.);
#4983=ORIENTED_EDGE('',*,*,#3830,.F.);
#4984=ORIENTED_EDGE('',*,*,#3754,.T.);
#4985=ORIENTED_EDGE('',*,*,#3835,.T.);
#4986=ORIENTED_EDGE('',*,*,#3845,.T.);
#4987=ORIENTED_EDGE('',*,*,#3839,.T.);
#4988=ORIENTED_EDGE('',*,*,#3846,.T.);
#4989=ORIENTED_EDGE('',*,*,#3767,.F.);
#4990=ORIENTED_EDGE('',*,*,#3766,.T.);
#4991=ORIENTED_EDGE('',*,*,#3761,.F.);
#4992=ORIENTED_EDGE('',*,*,#3845,.F.);
#4993=ORIENTED_EDGE('',*,*,#3838,.F.);
#4994=ORIENTED_EDGE('',*,*,#3819,.F.);
#4995=ORIENTED_EDGE('',*,*,#3840,.F.);
#4996=ORIENTED_EDGE('',*,*,#3827,.F.);
#4997=ORIENTED_EDGE('',*,*,#3837,.F.);
#4998=ORIENTED_EDGE('',*,*,#3844,.F.);
#4999=ORIENTED_EDGE('',*,*,#3798,.F.);
#5000=ORIENTED_EDGE('',*,*,#3843,.F.);
#5001=ORIENTED_EDGE('',*,*,#3832,.F.);
#5002=ORIENTED_EDGE('',*,*,#3828,.F.);
#5003=ORIENTED_EDGE('',*,*,#3800,.F.);
#5004=ORIENTED_EDGE('',*,*,#3823,.F.);
#5005=ORIENTED_EDGE('',*,*,#3831,.F.);
#5006=ORIENTED_EDGE('',*,*,#3846,.F.);
#5007=ORIENTED_EDGE('',*,*,#3841,.F.);
#5008=ORIENTED_EDGE('',*,*,#3748,.F.);
#5009=ORIENTED_EDGE('',*,*,#3842,.F.);
#5010=ORIENTED_EDGE('',*,*,#3796,.F.);
#5011=ORIENTED_EDGE('',*,*,#3834,.F.);
#5012=ORIENTED_EDGE('',*,*,#3793,.F.);
#5013=ORIENTED_EDGE('',*,*,#3791,.F.);
#5014=ORIENTED_EDGE('',*,*,#3847,.T.);
#5015=ORIENTED_EDGE('',*,*,#3848,.T.);
#5016=ORIENTED_EDGE('',*,*,#3849,.T.);
#5017=ORIENTED_EDGE('',*,*,#3850,.T.);
#5018=ORIENTED_EDGE('',*,*,#3851,.T.);
#5019=ORIENTED_EDGE('',*,*,#3852,.T.);
#5020=ORIENTED_EDGE('',*,*,#3847,.F.);
#5021=ORIENTED_EDGE('',*,*,#3853,.T.);
#5022=ORIENTED_EDGE('',*,*,#3854,.F.);
#5023=ORIENTED_EDGE('',*,*,#3807,.T.);
#5024=ORIENTED_EDGE('',*,*,#3760,.F.);
#5025=ORIENTED_EDGE('',*,*,#3855,.T.);
#5026=ORIENTED_EDGE('',*,*,#3856,.T.);
#5027=ORIENTED_EDGE('',*,*,#3851,.F.);
#5028=ORIENTED_EDGE('',*,*,#3806,.T.);
#5029=ORIENTED_EDGE('',*,*,#3849,.F.);
#5030=ORIENTED_EDGE('',*,*,#3857,.T.);
#5031=ORIENTED_EDGE('',*,*,#3855,.F.);
#5032=ORIENTED_EDGE('',*,*,#3809,.T.);
#5033=ORIENTED_EDGE('',*,*,#3858,.T.);
#5034=ORIENTED_EDGE('',*,*,#3859,.T.);
#5035=ORIENTED_EDGE('',*,*,#3758,.F.);
#5036=ORIENTED_EDGE('',*,*,#3854,.T.);
#5037=ORIENTED_EDGE('',*,*,#3860,.T.);
#5038=ORIENTED_EDGE('',*,*,#3858,.F.);
#5039=ORIENTED_EDGE('',*,*,#3808,.T.);
#5040=ORIENTED_EDGE('',*,*,#3852,.F.);
#5041=ORIENTED_EDGE('',*,*,#3856,.F.);
#5042=ORIENTED_EDGE('',*,*,#3857,.F.);
#5043=ORIENTED_EDGE('',*,*,#3848,.F.);
#5044=ORIENTED_EDGE('',*,*,#3859,.F.);
#5045=ORIENTED_EDGE('',*,*,#3860,.F.);
#5046=ORIENTED_EDGE('',*,*,#3853,.F.);
#5047=ORIENTED_EDGE('',*,*,#3850,.F.);
#6512=ADVANCED_FACE('',(#1860),#1669,.F.);
#6513=ADVANCED_FACE('',(#1861),#1670,.F.);
#6514=ADVANCED_FACE('',(#1862),#1671,.T.);
#6515=ADVANCED_FACE('',(#1863),#1672,.T.);
#6516=ADVANCED_FACE('',(#1864),#1673,.T.);
#6517=ADVANCED_FACE('',(#1865),#1674,.F.);
#6518=ADVANCED_FACE('',(#1866),#1675,.F.);
#6519=ADVANCED_FACE('',(#1867,#290,#291),#117,.T.);
#6520=ADVANCED_FACE('',(#1868),#416,.F.);
#6521=ADVANCED_FACE('',(#1869),#417,.F.);
#6522=ADVANCED_FACE('',(#1870),#418,.F.);
#6523=ADVANCED_FACE('',(#1871),#419,.T.);
#6524=ADVANCED_FACE('',(#1872),#118,.T.);
#6525=ADVANCED_FACE('',(#1873),#1676,.F.);
#6526=ADVANCED_FACE('',(#1874,#292),#1677,.T.);
#6527=ADVANCED_FACE('',(#1875),#420,.T.);
#6528=ADVANCED_FACE('',(#1876,#293),#421,.T.);
#6529=ADVANCED_FACE('',(#1877,#294),#422,.T.);
#6530=ADVANCED_FACE('',(#1878),#423,.F.);
#6531=ADVANCED_FACE('',(#1879),#424,.F.);
#6532=ADVANCED_FACE('',(#1880,#295),#425,.F.);
#6533=ADVANCED_FACE('',(#1881),#426,.F.);
#6534=ADVANCED_FACE('',(#1882,#296),#427,.F.);
#6535=ADVANCED_FACE('',(#1883),#428,.F.);
#6536=ADVANCED_FACE('',(#1884),#429,.F.);
#6537=ADVANCED_FACE('',(#1885),#430,.T.);
#6538=ADVANCED_FACE('',(#1886),#431,.F.);
#6539=ADVANCED_FACE('',(#1887,#297),#432,.F.);
#6540=ADVANCED_FACE('',(#1888,#298),#433,.F.);
#6541=ADVANCED_FACE('',(#1889),#434,.T.);
#6542=ADVANCED_FACE('',(#1890),#435,.F.);
#6543=ADVANCED_FACE('',(#1891),#1678,.T.);
#6544=ADVANCED_FACE('',(#1892),#1679,.T.);
#6545=ADVANCED_FACE('',(#1893),#1680,.T.);
#6546=ADVANCED_FACE('',(#1894),#1681,.T.);
#6547=ADVANCED_FACE('',(#1895),#1682,.T.);
#6548=ADVANCED_FACE('',(#1896),#436,.F.);
#6549=ADVANCED_FACE('',(#1897,#299),#437,.T.);
#6550=ADVANCED_FACE('',(#1898),#438,.T.);
#6551=ADVANCED_FACE('',(#1899,#300),#439,.T.);
#6552=ADVANCED_FACE('',(#1900),#440,.T.);
#6553=ADVANCED_FACE('',(#1901),#1683,.T.);
#6554=ADVANCED_FACE('',(#1902),#1684,.T.);
#6844=CLOSED_SHELL('',(#6512,#6513,#6514,#6515,#6516,#6517,#6518,#6519,
#6520,#6521,#6522,#6523,#6524,#6525,#6526,#6527,#6528,#6529,#6530,#6531,
#6532,#6533,#6534,#6535,#6536,#6537,#6538,#6539,#6540,#6541,#6542,#6543,
#6544,#6545,#6546,#6547,#6548,#6549,#6550,#6551,#6552,#6553,#6554));
#7193=AXIS2_PLACEMENT_3D('',#10156,#8157,#8158);
#7194=AXIS2_PLACEMENT_3D('',#10157,#8159,#8160);
#7195=AXIS2_PLACEMENT_3D('',#10179,#8161,#8162);
#7196=AXIS2_PLACEMENT_3D('',#10183,#8164,#8165);
#7197=AXIS2_PLACEMENT_3D('',#10187,#8167,#8168);
#7198=AXIS2_PLACEMENT_3D('',#10191,#8170,#8171);
#7199=AXIS2_PLACEMENT_3D('',#10194,#8173,#8174);
#7200=AXIS2_PLACEMENT_3D('',#10195,#8175,#8176);
#7201=AXIS2_PLACEMENT_3D('',#10197,#8177,#8178);
#7202=AXIS2_PLACEMENT_3D('',#10200,#8180,#8181);
#7203=AXIS2_PLACEMENT_3D('',#10201,#8182,#8183);
#7204=AXIS2_PLACEMENT_3D('',#10203,#8184,#8185);
#7205=AXIS2_PLACEMENT_3D('',#10206,#8187,#8188);
#7206=AXIS2_PLACEMENT_3D('',#10207,#8189,#8190);
#7207=AXIS2_PLACEMENT_3D('',#10209,#8191,#8192);
#7208=AXIS2_PLACEMENT_3D('',#10212,#8194,#8195);
#7209=AXIS2_PLACEMENT_3D('',#10213,#8196,#8197);
#7210=AXIS2_PLACEMENT_3D('',#10215,#8198,#8199);
#7211=AXIS2_PLACEMENT_3D('',#10218,#8201,#8202);
#7212=AXIS2_PLACEMENT_3D('',#10219,#8203,#8204);
#7213=AXIS2_PLACEMENT_3D('',#10221,#8205,#8206);
#7214=AXIS2_PLACEMENT_3D('',#10262,#8208,#8209);
#7215=AXIS2_PLACEMENT_3D('',#10285,#8211,#8212);
#7216=AXIS2_PLACEMENT_3D('',#10305,#8213,#8214);
#7217=AXIS2_PLACEMENT_3D('',#10308,#8215,#8216);
#7218=AXIS2_PLACEMENT_3D('',#10342,#8217,#8218);
#7219=AXIS2_PLACEMENT_3D('',#10399,#8220,#8221);
#7220=AXIS2_PLACEMENT_3D('',#10431,#8222,#8223);
#7221=AXIS2_PLACEMENT_3D('',#10435,#8226,#8227);
#7222=AXIS2_PLACEMENT_3D('',#10438,#8229,#8230);
#7223=AXIS2_PLACEMENT_3D('',#10439,#8231,#8232);
#7224=AXIS2_PLACEMENT_3D('',#10444,#8235,#8236);
#7225=AXIS2_PLACEMENT_3D('',#10445,#8237,#8238);
#7226=AXIS2_PLACEMENT_3D('',#10454,#8243,#8244);
#7227=AXIS2_PLACEMENT_3D('',#10455,#8245,#8246);
#7228=AXIS2_PLACEMENT_3D('',#10466,#8247,#8248);
#7229=AXIS2_PLACEMENT_3D('',#10470,#8250,#8251);
#7230=AXIS2_PLACEMENT_3D('',#10471,#8252,#8253);
#7231=AXIS2_PLACEMENT_3D('',#10472,#8254,#8255);
#7232=AXIS2_PLACEMENT_3D('',#10477,#8257,#8258);
#7233=AXIS2_PLACEMENT_3D('',#10480,#8260,#8261);
#7234=AXIS2_PLACEMENT_3D('',#10481,#8262,#8263);
#7235=AXIS2_PLACEMENT_3D('',#10487,#8267,#8268);
#7236=AXIS2_PLACEMENT_3D('',#10489,#8270,#8271);
#7237=AXIS2_PLACEMENT_3D('',#10491,#8273,#8274);
#7238=AXIS2_PLACEMENT_3D('',#10492,#8275,#8276);
#7239=AXIS2_PLACEMENT_3D('',#10498,#8280,#8281);
#7240=AXIS2_PLACEMENT_3D('',#10503,#8283,#8284);
#7241=AXIS2_PLACEMENT_3D('',#10509,#8288,#8289);
#7242=AXIS2_PLACEMENT_3D('',#10510,#8290,#8291);
#7243=AXIS2_PLACEMENT_3D('',#10514,#8294,#8295);
#7244=AXIS2_PLACEMENT_3D('',#10517,#8297,#8298);
#7245=AXIS2_PLACEMENT_3D('',#10519,#8299,#8300);
#7246=AXIS2_PLACEMENT_3D('',#10521,#8302,#8303);
#7247=AXIS2_PLACEMENT_3D('',#10529,#8309,#8310);
#7248=AXIS2_PLACEMENT_3D('',#10536,#8315,#8316);
#7249=AXIS2_PLACEMENT_3D('',#10542,#8320,#8321);
#7250=AXIS2_PLACEMENT_3D('',#10544,#8323,#8324);
#7251=AXIS2_PLACEMENT_3D('',#10545,#8325,#8326);
#7252=AXIS2_PLACEMENT_3D('',#10546,#8327,#8328);
#7253=AXIS2_PLACEMENT_3D('',#10547,#8329,#8330);
#7254=AXIS2_PLACEMENT_3D('',#10548,#8331,#8332);
#7255=AXIS2_PLACEMENT_3D('',#10549,#8333,#8334);
#7256=AXIS2_PLACEMENT_3D('',#10550,#8335,#8336);
#7257=AXIS2_PLACEMENT_3D('',#10551,#8337,#8338);
#7258=AXIS2_PLACEMENT_3D('',#10552,#8339,#8340);
#7259=AXIS2_PLACEMENT_3D('',#10553,#8341,#8342);
#7260=AXIS2_PLACEMENT_3D('',#10554,#8343,#8344);
#7261=AXIS2_PLACEMENT_3D('',#10555,#8345,#8346);
#7262=AXIS2_PLACEMENT_3D('',#10556,#8347,#8348);
#7263=AXIS2_PLACEMENT_3D('',#10557,#8349,#8350);
#7264=AXIS2_PLACEMENT_3D('',#10566,#8355,#8356);
#7265=AXIS2_PLACEMENT_3D('',#10569,#8358,#8359);
#7266=AXIS2_PLACEMENT_3D('',#10571,#8360,#8361);
#7267=AXIS2_PLACEMENT_3D('',#10573,#8363,#8364);
#7268=AXIS2_PLACEMENT_3D('',#10577,#8367,#8368);
#7269=AXIS2_PLACEMENT_3D('',#10578,#8369,#8370);
#7270=AXIS2_PLACEMENT_3D('',#10581,#8372,#8373);
#7271=AXIS2_PLACEMENT_3D('',#10582,#8374,#8375);
#7272=AXIS2_PLACEMENT_3D('',#10584,#8377,#8378);
#7273=AXIS2_PLACEMENT_3D('',#10585,#8379,#8380);
#8157=DIRECTION('axis',(0.,0.,1.));
#8158=DIRECTION('refdir',(1.,0.,0.));
#8159=DIRECTION('center_axis',(0.,0.,1.));
#8160=DIRECTION('ref_axis',(1.,0.,0.));
#8161=DIRECTION('center_axis',(0.707106781186558,-5.01171544695272E-14,
0.707106781186537));
#8162=DIRECTION('ref_axis',(0.707106781186537,1.30563837326012E-11,-0.707106781186558));
#8163=DIRECTION('',(0.,0.,1.));
#8164=DIRECTION('center_axis',(-0.707106781186548,-3.66800410274155E-14,
0.707106781186547));
#8165=DIRECTION('ref_axis',(0.707106781186547,-1.32695584283249E-13,0.707106781186548));
#8166=DIRECTION('',(0.,0.,1.));
#8167=DIRECTION('center_axis',(0.707106781186548,-2.49447284670762E-16,
-0.707106781186547));
#8168=DIRECTION('ref_axis',(0.707106781186547,3.43199962798826E-15,0.707106781186548));
#8169=DIRECTION('',(0.,0.,1.));
#8170=DIRECTION('center_axis',(-0.707106781186548,-5.83546107254331E-15,
0.707106781186547));
#8171=DIRECTION('ref_axis',(0.707106781186547,-8.39541658988548E-14,0.707106781186548));
#8172=DIRECTION('',(0.,0.,-1.));
#8173=DIRECTION('center_axis',(0.70710678118654,-3.75878658521447E-14,0.707106781186555));
#8174=DIRECTION('ref_axis',(0.707106781186555,-7.50458522379288E-12,-0.70710678118654));
#8175=DIRECTION('center_axis',(0.,-1.,0.));
#8176=DIRECTION('ref_axis',(0.,0.,-1.));
#8177=DIRECTION('center_axis',(0.,1.,0.));
#8178=DIRECTION('ref_axis',(0.,0.,1.));
#8179=DIRECTION('',(0.,-1.,0.));
#8180=DIRECTION('center_axis',(0.,-1.,0.));
#8181=DIRECTION('ref_axis',(0.,0.,-1.));
#8182=DIRECTION('center_axis',(0.,1.,0.));
#8183=DIRECTION('ref_axis',(0.,0.,1.));
#8184=DIRECTION('center_axis',(0.,-1.,0.));
#8185=DIRECTION('ref_axis',(0.,0.,-1.));
#8186=DIRECTION('',(0.,-1.,0.));
#8187=DIRECTION('center_axis',(0.,1.,0.));
#8188=DIRECTION('ref_axis',(0.,0.,-1.));
#8189=DIRECTION('center_axis',(0.,1.,0.));
#8190=DIRECTION('ref_axis',(0.,0.,1.));
#8191=DIRECTION('center_axis',(0.,-1.,0.));
#8192=DIRECTION('ref_axis',(0.,0.,1.));
#8193=DIRECTION('',(0.,-1.,0.));
#8194=DIRECTION('center_axis',(0.,-1.,0.));
#8195=DIRECTION('ref_axis',(0.,0.,-1.));
#8196=DIRECTION('center_axis',(0.,1.,0.));
#8197=DIRECTION('ref_axis',(0.,0.,1.));
#8198=DIRECTION('center_axis',(0.,-1.,0.));
#8199=DIRECTION('ref_axis',(0.,0.,1.));
#8200=DIRECTION('',(0.,-1.,0.));
#8201=DIRECTION('center_axis',(0.,1.,0.));
#8202=DIRECTION('ref_axis',(0.,0.,-1.));
#8203=DIRECTION('center_axis',(0.,-1.,0.));
#8204=DIRECTION('ref_axis',(0.,0.,-1.));
#8205=DIRECTION('center_axis',(0.,-1.,-1.24352412568707E-16));
#8206=DIRECTION('ref_axis',(0.,-1.24352412568707E-16,1.));
#8207=DIRECTION('',(0.,-1.,0.));
#8208=DIRECTION('center_axis',(0.,-1.,0.));
#8209=DIRECTION('ref_axis',(0.,0.,-1.));
#8210=DIRECTION('',(0.,-1.,0.));
#8211=DIRECTION('center_axis',(0.,1.,1.24352412568707E-16));
#8212=DIRECTION('ref_axis',(0.,1.24352412568707E-16,-1.));
#8213=DIRECTION('center_axis',(0.,0.,-1.));
#8214=DIRECTION('ref_axis',(1.,0.,0.));
#8215=DIRECTION('center_axis',(0.,1.15648231731787E-16,-1.));
#8216=DIRECTION('ref_axis',(0.,1.,1.15648231731787E-16));
#8217=DIRECTION('center_axis',(0.,0.,1.));
#8218=DIRECTION('ref_axis',(-1.,0.,0.));
#8219=DIRECTION('',(0.0174524064372835,-2.1373033680838E-18,0.999847695156391));
#8220=DIRECTION('center_axis',(0.,0.,1.));
#8221=DIRECTION('ref_axis',(-1.,0.,0.));
#8222=DIRECTION('center_axis',(0.707106781186548,0.,0.707106781186548));
#8223=DIRECTION('ref_axis',(0.707106781186548,0.,-0.707106781186548));
#8224=DIRECTION('',(-0.707106781186547,0.,0.707106781186547));
#8225=DIRECTION('',(0.,-1.,0.));
#8226=DIRECTION('center_axis',(0.,-1.,0.));
#8227=DIRECTION('ref_axis',(0.,0.,-1.));
#8228=DIRECTION('',(0.707106781186548,0.,0.707106781186548));
#8229=DIRECTION('center_axis',(0.,-1.,0.));
#8230=DIRECTION('ref_axis',(0.,0.,-1.));
#8231=DIRECTION('center_axis',(0.,1.,0.));
#8232=DIRECTION('ref_axis',(0.,0.,1.));
#8233=DIRECTION('',(-0.707106781186547,0.,0.707106781186547));
#8234=DIRECTION('',(-0.707106781186548,0.,-0.707106781186548));
#8235=DIRECTION('center_axis',(0.,1.,0.));
#8236=DIRECTION('ref_axis',(0.,0.,1.));
#8237=DIRECTION('center_axis',(-0.707106781186547,0.,-0.707106781186548));
#8238=DIRECTION('ref_axis',(-0.707106781186548,0.,0.707106781186547));
#8239=DIRECTION('',(-0.707106781186548,0.,0.707106781186547));
#8240=DIRECTION('',(0.,1.,0.));
#8241=DIRECTION('',(-0.707106781186548,0.,0.707106781186547));
#8242=DIRECTION('',(0.,-1.,0.));
#8243=DIRECTION('center_axis',(0.,0.,-1.));
#8244=DIRECTION('ref_axis',(-1.,-1.22464679914735E-16,0.));
#8245=DIRECTION('center_axis',(0.,0.,-1.));
#8246=DIRECTION('ref_axis',(1.,1.77635683940025E-15,0.));
#8247=DIRECTION('center_axis',(0.,-1.,0.));
#8248=DIRECTION('ref_axis',(-0.185273532463833,0.,0.982686988907644));
#8249=DIRECTION('',(0.,1.,0.));
#8250=DIRECTION('center_axis',(0.,1.,1.24352412568707E-16));
#8251=DIRECTION('ref_axis',(0.,-1.24352412568707E-16,1.));
#8252=DIRECTION('center_axis',(0.,-1.,-1.24352412568707E-16));
#8253=DIRECTION('ref_axis',(0.,1.24352412568707E-16,-1.));
#8254=DIRECTION('center_axis',(0.,-1.,0.));
#8255=DIRECTION('ref_axis',(3.0760962761356E-5,0.,0.999999999526882));
#8256=DIRECTION('',(0.,1.,0.));
#8257=DIRECTION('center_axis',(0.,1.,0.));
#8258=DIRECTION('ref_axis',(0.,0.,-1.));
#8259=DIRECTION('',(0.,-1.,0.));
#8260=DIRECTION('center_axis',(0.,-1.,0.));
#8261=DIRECTION('ref_axis',(0.,0.,1.));
#8262=DIRECTION('center_axis',(0.,1.15648231731787E-16,-1.));
#8263=DIRECTION('ref_axis',(0.,1.,1.15648231731787E-16));
#8264=DIRECTION('',(-1.,0.,0.));
#8265=DIRECTION('',(0.,-1.,-1.15648231731787E-16));
#8266=DIRECTION('',(-1.,0.,0.));
#8267=DIRECTION('center_axis',(0.,1.,1.24352412568707E-16));
#8268=DIRECTION('ref_axis',(0.,-1.24352412568707E-16,1.));
#8269=DIRECTION('',(0.,1.24352412568707E-16,-1.));
#8270=DIRECTION('center_axis',(0.,-1.,-1.24352412568707E-16));
#8271=DIRECTION('ref_axis',(0.,1.24352412568707E-16,-1.));
#8272=DIRECTION('',(0.,-1.24352412568707E-16,1.));
#8273=DIRECTION('center_axis',(-1.,0.,0.));
#8274=DIRECTION('ref_axis',(0.,0.,1.));
#8275=DIRECTION('center_axis',(0.,0.,1.));
#8276=DIRECTION('ref_axis',(1.,0.,0.));
#8277=DIRECTION('',(-1.,0.,0.));
#8278=DIRECTION('',(0.,1.,0.));
#8279=DIRECTION('',(-1.,0.,0.));
#8280=DIRECTION('center_axis',(0.,-1.,0.));
#8281=DIRECTION('ref_axis',(0.,0.,-1.));
#8282=DIRECTION('',(0.707106781186548,0.,-0.707106781186547));
#8283=DIRECTION('center_axis',(0.,1.,0.));
#8284=DIRECTION('ref_axis',(0.,0.,-1.));
#8285=DIRECTION('',(0.707106781186548,0.,0.707106781186548));
#8286=DIRECTION('',(-1.,0.,0.));
#8287=DIRECTION('',(0.707106781186548,0.,0.707106781186548));
#8288=DIRECTION('center_axis',(0.,1.,0.));
#8289=DIRECTION('ref_axis',(-3.46944695195361E-15,0.,-1.));
#8290=DIRECTION('center_axis',(0.,0.,-1.));
#8291=DIRECTION('ref_axis',(-1.,0.,0.));
#8292=DIRECTION('',(0.,-1.,0.));
#8293=DIRECTION('',(-1.,0.,0.));
#8294=DIRECTION('center_axis',(0.,1.,0.));
#8295=DIRECTION('ref_axis',(0.,0.,1.));
#8296=DIRECTION('',(0.707106781186548,0.,0.707106781186548));
#8297=DIRECTION('center_axis',(0.,-1.,0.));
#8298=DIRECTION('ref_axis',(3.46944695195361E-15,0.,1.));
#8299=DIRECTION('center_axis',(0.,-1.,0.));
#8300=DIRECTION('ref_axis',(-3.46944695195361E-15,0.,1.));
#8301=DIRECTION('',(0.707106781186548,0.,0.707106781186548));
#8302=DIRECTION('center_axis',(-0.707106781186548,0.,0.707106781186547));
#8303=DIRECTION('ref_axis',(0.707106781186547,0.,0.707106781186548));
#8304=DIRECTION('',(-0.707106781186548,0.,-0.707106781186548));
#8305=DIRECTION('',(0.,1.,0.));
#8306=DIRECTION('',(0.,1.,0.));
#8307=DIRECTION('',(0.707106781186548,0.,0.707106781186548));
#8308=DIRECTION('',(0.,1.,0.));
#8309=DIRECTION('center_axis',(0.707106781186548,0.,-0.707106781186547));
#8310=DIRECTION('ref_axis',(-0.707106781186547,0.,-0.707106781186548));
#8311=DIRECTION('',(-0.707106781186548,0.,-0.707106781186548));
#8312=DIRECTION('',(0.707106781186548,0.,0.707106781186548));
#8313=DIRECTION('',(0.,-1.,0.));
#8314=DIRECTION('',(0.,-1.,0.));
#8315=DIRECTION('center_axis',(-0.707106781186547,0.,-0.707106781186548));
#8316=DIRECTION('ref_axis',(-0.707106781186548,0.,0.707106781186547));
#8317=DIRECTION('',(0.707106781186548,0.,-0.707106781186547));
#8318=DIRECTION('',(0.,1.,0.));
#8319=DIRECTION('',(0.,-1.,0.));
#8320=DIRECTION('center_axis',(0.707106781186548,0.,0.707106781186548));
#8321=DIRECTION('ref_axis',(0.707106781186548,0.,-0.707106781186548));
#8322=DIRECTION('',(0.,-1.,0.));
#8323=DIRECTION('center_axis',(0.,-1.,0.));
#8324=DIRECTION('ref_axis',(0.,0.,-1.));
#8325=DIRECTION('center_axis',(0.,1.,0.));
#8326=DIRECTION('ref_axis',(-3.46944695195361E-15,0.,-1.));
#8327=DIRECTION('center_axis',(0.,1.,0.));
#8328=DIRECTION('ref_axis',(0.,0.,-1.));
#8329=DIRECTION('center_axis',(0.,1.,0.));
#8330=DIRECTION('ref_axis',(0.,0.,1.));
#8331=DIRECTION('center_axis',(0.,-1.,0.));
#8332=DIRECTION('ref_axis',(0.,0.,1.));
#8333=DIRECTION('center_axis',(0.,-1.,0.));
#8334=DIRECTION('ref_axis',(-3.46944695195361E-15,0.,1.));
#8335=DIRECTION('center_axis',(0.,-1.,0.));
#8336=DIRECTION('ref_axis',(0.,0.,-1.));
#8337=DIRECTION('center_axis',(0.,-1.,0.));
#8338=DIRECTION('ref_axis',(0.,0.,-1.));
#8339=DIRECTION('center_axis',(0.,-1.,0.));
#8340=DIRECTION('ref_axis',(0.,0.,-1.));
#8341=DIRECTION('center_axis',(0.,-1.,0.));
#8342=DIRECTION('ref_axis',(0.,0.,-1.));
#8343=DIRECTION('center_axis',(0.,1.,0.));
#8344=DIRECTION('ref_axis',(1.45473230946492E-15,0.,-1.));
#8345=DIRECTION('center_axis',(0.,1.,0.));
#8346=DIRECTION('ref_axis',(1.45473230946492E-15,0.,-1.));
#8347=DIRECTION('center_axis',(0.,1.,0.));
#8348=DIRECTION('ref_axis',(-1.22464679914735E-16,0.,-1.));
#8349=DIRECTION('center_axis',(0.,0.,-1.));
#8350=DIRECTION('ref_axis',(-1.,0.,0.));
#8351=DIRECTION('',(1.,0.,0.));
#8352=DIRECTION('',(0.,1.,0.));
#8353=DIRECTION('',(-1.,0.,0.));
#8354=DIRECTION('',(0.,-1.,0.));
#8355=DIRECTION('center_axis',(0.,-1.,0.));
#8356=DIRECTION('ref_axis',(0.,0.,-1.));
#8357=DIRECTION('',(0.,0.,1.));
#8358=DIRECTION('center_axis',(0.,-1.,0.));
#8359=DIRECTION('ref_axis',(0.,0.,-1.));
#8360=DIRECTION('center_axis',(0.,-1.,0.));
#8361=DIRECTION('ref_axis',(0.,0.,-1.));
#8362=DIRECTION('',(0.,0.,1.));
#8363=DIRECTION('center_axis',(1.,0.,0.));
#8364=DIRECTION('ref_axis',(0.,0.,-1.));
#8365=DIRECTION('',(0.,0.,1.));
#8366=DIRECTION('',(0.,-1.,0.));
#8367=DIRECTION('center_axis',(0.,1.,0.));
#8368=DIRECTION('ref_axis',(0.,0.,1.));
#8369=DIRECTION('center_axis',(0.,1.,0.));
#8370=DIRECTION('ref_axis',(0.,0.,1.));
#8371=DIRECTION('',(0.,0.,1.));
#8372=DIRECTION('center_axis',(0.,1.,0.));
#8373=DIRECTION('ref_axis',(0.,0.,1.));
#8374=DIRECTION('center_axis',(-1.,0.,0.));
#8375=DIRECTION('ref_axis',(0.,0.,1.));
#8376=DIRECTION('',(0.,1.,0.));
#8377=DIRECTION('center_axis',(0.,-1.,0.));
#8378=DIRECTION('ref_axis',(0.,0.,-1.));
#8379=DIRECTION('center_axis',(0.,1.,0.));
#8380=DIRECTION('ref_axis',(0.,0.,1.));
#10156=CARTESIAN_POINT('',(0.,0.,0.));
#10157=CARTESIAN_POINT('Origin',(-16.3495307931818,0.,-13.5491970462687));
#10158=CARTESIAN_POINT('',(-15.1213202922933,2.27257763076018,-0.256303827455242));
#10159=CARTESIAN_POINT('',(-15.1213202922933,-2.27257763076018,-0.256303827455243));
#10160=CARTESIAN_POINT('Ctrl Pts',(-15.1213202922914,2.27257763075913,-0.256303827457184));
#10161=CARTESIAN_POINT('Ctrl Pts',(-15.0515142687323,2.23485109064003,-0.326109851015821));
#10162=CARTESIAN_POINT('Ctrl Pts',(-14.9635999263237,2.18198234976026,-0.389326304386628));
#10163=CARTESIAN_POINT('Ctrl Pts',(-14.7279251205928,2.02003601855949,-0.515618311313952));
#10164=CARTESIAN_POINT('Ctrl Pts',(-14.5398271293955,1.85535578506882,-0.550855368407477));
#10165=CARTESIAN_POINT('Ctrl Pts',(-14.2038906955615,1.46968867782391,-0.54663177315069));
#10166=CARTESIAN_POINT('Ctrl Pts',(-14.0399657872398,1.1984002224899,-0.484906409913535));
#10167=CARTESIAN_POINT('Ctrl Pts',(-13.8212117604045,0.614696166914028,
-0.364038582843676));
#10168=CARTESIAN_POINT('Ctrl Pts',(-13.76629442724,0.301085199472153,-0.310906216990201));
#10169=CARTESIAN_POINT('Ctrl Pts',(-13.76629442724,-0.301085199472153,-0.310906216990201));
#10170=CARTESIAN_POINT('Ctrl Pts',(-13.8212117604045,-0.614696166914028,
-0.364038582843676));
#10171=CARTESIAN_POINT('Ctrl Pts',(-14.0399657872398,-1.1984002224899,-0.484906409913535));
#10172=CARTESIAN_POINT('Ctrl Pts',(-14.2038906955615,-1.46968867782391,
-0.54663177315069));
#10173=CARTESIAN_POINT('Ctrl Pts',(-14.5398271293955,-1.85535578506882,
-0.550855368407477));
#10174=CARTESIAN_POINT('Ctrl Pts',(-14.7279251205928,-2.02003601855949,
-0.515618311313952));
#10175=CARTESIAN_POINT('Ctrl Pts',(-14.9635999263244,-2.18198234976076,
-0.389326304386245));
#10176=CARTESIAN_POINT('Ctrl Pts',(-15.0515142687339,-2.23485109064098,
-0.326109851014598));
#10177=CARTESIAN_POINT('Ctrl Pts',(-15.1213202922933,-2.27257763076018,
-0.256303827455241));
#10178=CARTESIAN_POINT('',(-15.69906163763,-2.5,0.321437517881415));
#10179=CARTESIAN_POINT('Origin',(-16.3495307931561,-6.40168473786673E-11,
0.971906673407791));
#10180=CARTESIAN_POINT('',(-15.69906163763,-2.5,-2.248258735165));
#10181=CARTESIAN_POINT('',(-15.69906163763,-2.5,-13.5491970462687));
#10182=CARTESIAN_POINT('',(-16.9999999487337,-2.5,-3.5491970462687));
#10183=CARTESIAN_POINT('Origin',(-16.3495307931821,1.13797860024079E-12,
-2.89872789071702));
#10184=CARTESIAN_POINT('',(-16.9999999487337,-2.5,2.4508029537313));
#10185=CARTESIAN_POINT('',(-16.9999999487337,-2.5,-13.5491970462687));
#10186=CARTESIAN_POINT('',(-16.9999999487337,2.5,2.4508029537313));
#10187=CARTESIAN_POINT('Origin',(-16.3495307931818,-1.27675647831893E-14,
3.10127210928315));
#10188=CARTESIAN_POINT('',(-16.9999999487337,2.5,-3.5491970462687));
#10189=CARTESIAN_POINT('',(-16.9999999487337,2.5,-13.5491970462687));
#10190=CARTESIAN_POINT('',(-15.69906163763,2.5,-2.248258735165));
#10191=CARTESIAN_POINT('Origin',(-16.3495307931817,-2.70228284193763E-12,
-2.89872789071671));
#10192=CARTESIAN_POINT('',(-15.69906163763,2.5,0.321437517881415));
#10193=CARTESIAN_POINT('',(-15.69906163763,2.5,-13.5491970462687));
#10194=CARTESIAN_POINT('Origin',(-16.3495307931675,4.20433132752862E-11,
0.971906673418779));
#10195=CARTESIAN_POINT('Origin',(-0.362549034825799,5.5798767903013,40.6388167522632));
#10196=CARTESIAN_POINT('',(-0.362549034825799,4.4201232096987,42.1388167522632));
#10197=CARTESIAN_POINT('Origin',(-0.362549034825799,4.4201232096987,40.6388167522632));
#10198=CARTESIAN_POINT('',(-0.362549034825799,-4.4201232096987,42.1388167522632));
#10199=CARTESIAN_POINT('',(-0.362549034825799,5.5798767903013,42.1388167522632));
#10200=CARTESIAN_POINT('Origin',(-0.362549034825799,-4.4201232096987,40.6388167522632));
#10201=CARTESIAN_POINT('Origin',(-18.0355338546664,-5.4201232096987,-1.58473095220143));
#10202=CARTESIAN_POINT('',(-18.0355338546664,5.4198767903013,-2.58473095220143));
#10203=CARTESIAN_POINT('Origin',(-18.0355338546664,5.4198767903013,-1.58473095220143));
#10204=CARTESIAN_POINT('',(-18.0355338546664,4.4201232096987,-2.58473095220143));
#10205=CARTESIAN_POINT('',(-18.0355338546664,-5.4201232096987,-2.58473095220143));
#10206=CARTESIAN_POINT('Origin',(-18.0355338546664,4.4201232096987,-1.58473095220143));
#10207=CARTESIAN_POINT('Origin',(-18.0355338546664,-5.4201232096987,-1.58473095220143));
#10208=CARTESIAN_POINT('',(-18.0355338546664,-4.4201232096987,-2.58473095220143));
#10209=CARTESIAN_POINT('Origin',(-18.0355338546664,-4.4201232096987,-1.58473095220143));
#10210=CARTESIAN_POINT('',(-18.0355338546664,-5.4201232096987,-2.58473095220143));
#10211=CARTESIAN_POINT('',(-18.0355338546664,-5.4201232096987,-2.58473095220143));
#10212=CARTESIAN_POINT('Origin',(-18.0355338546664,-5.4201232096987,-1.58473095220143));
#10213=CARTESIAN_POINT('Origin',(-18.0355338546664,-5.4201232096987,-1.58473095220143));
#10214=CARTESIAN_POINT('',(-18.0355338546664,2.5,-2.58473095220143));
#10215=CARTESIAN_POINT('Origin',(-18.0355338546664,2.5,-1.58473095220143));
#10216=CARTESIAN_POINT('',(-18.0355338546664,-2.5,-2.58473095220143));
#10217=CARTESIAN_POINT('',(-18.0355338546664,-5.4201232096987,-2.58473095220143));
#10218=CARTESIAN_POINT('Origin',(-18.0355338546664,-2.5,-1.58473095220143));
#10219=CARTESIAN_POINT('Origin',(0.,18.,8.9205064589513));
#10220=CARTESIAN_POINT('',(-1.83697019872103E-16,-7.5,10.4205064589513));
#10221=CARTESIAN_POINT('Origin',(0.,-7.5,8.9205064589513));
#10222=CARTESIAN_POINT('',(-4.90834909410717E-16,-12.8181093831741,10.4205064589513));
#10223=CARTESIAN_POINT('',(-1.83697019872103E-16,18.,10.4205064589513));
#10224=CARTESIAN_POINT('',(1.27014494349635E-22,-12.8704745779587,7.4205064589513));
#10225=CARTESIAN_POINT('Ctrl Pts',(-6.59194920871187E-16,-12.8181093831741,
10.4205064589513));
#10226=CARTESIAN_POINT('Ctrl Pts',(-0.188255416016175,-12.8181093831741,
10.4205064589513));
#10227=CARTESIAN_POINT('Ctrl Pts',(-0.388988082274336,-12.8141939984886,
10.382902535549));
#10228=CARTESIAN_POINT('Ctrl Pts',(-0.758190528251416,-12.8003284816585,
10.2301098837158));
#10229=CARTESIAN_POINT('Ctrl Pts',(-0.92667197373005,-12.7906121431377,
10.114928217594));
#10230=CARTESIAN_POINT('Ctrl Pts',(-1.19277418140575,-12.7732022326273,
9.8492775803417));
#10231=CARTESIAN_POINT('Ctrl Pts',(-1.30822298061652,-12.7643815870671,
9.68105805060626));
#10232=CARTESIAN_POINT('Ctrl Pts',(-1.46164584377514,-12.7542036356865,
9.31226849459714));
#10233=CARTESIAN_POINT('Ctrl Pts',(-1.49961339720195,-12.7530891067545,
9.1116890996567));
#10234=CARTESIAN_POINT('Ctrl Pts',(-1.50038190415455,-12.7596246829664,
8.73468650392867));
#10235=CARTESIAN_POINT('Ctrl Pts',(-1.46294688463921,-12.7677413612085,
8.53336354542309));
#10236=CARTESIAN_POINT('Ctrl Pts',(-1.31017366956046,-12.7908167965405,
8.16318338701933));
#10237=CARTESIAN_POINT('Ctrl Pts',(-1.19484729740032,-12.8055313315293,
7.9943061245009));
#10238=CARTESIAN_POINT('Ctrl Pts',(-0.928670576176699,-12.8322493038568,
7.72758625806842));
#10239=CARTESIAN_POINT('Ctrl Pts',(-0.760025360862946,-12.8460029733389,
7.61189577191482));
#10240=CARTESIAN_POINT('Ctrl Pts',(-0.390125974594805,-12.8652326714021,
7.45834976030836));
#10241=CARTESIAN_POINT('Ctrl Pts',(-0.188854595603413,-12.8704745779587,
7.4205064589513));
#10242=CARTESIAN_POINT('Ctrl Pts',(-6.93889390390723E-17,-12.8704745779587,
7.4205064589513));
#10243=CARTESIAN_POINT('Ctrl Pts',(3.46944695195361E-17,-12.8704745779587,
7.4205064589513));
#10244=CARTESIAN_POINT('Ctrl Pts',(0.188854595603413,-12.8704745779587,
7.4205064589513));
#10245=CARTESIAN_POINT('Ctrl Pts',(0.390125974594805,-12.8652326714021,
7.45834976030836));
#10246=CARTESIAN_POINT('Ctrl Pts',(0.760025360862947,-12.8460029733389,
7.61189577191482));
#10247=CARTESIAN_POINT('Ctrl Pts',(0.928670576176699,-12.8322493038568,
7.72758625806842));
#10248=CARTESIAN_POINT('Ctrl Pts',(1.19484729740032,-12.8055313315293,7.9943061245009));
#10249=CARTESIAN_POINT('Ctrl Pts',(1.31017366956046,-12.7908167965405,8.16318338701932));
#10250=CARTESIAN_POINT('Ctrl Pts',(1.4629468846392,-12.7677413612085,8.53336354542309));
#10251=CARTESIAN_POINT('Ctrl Pts',(1.50038190415455,-12.7596246829664,8.73468650392867));
#10252=CARTESIAN_POINT('Ctrl Pts',(1.49999688350216,-12.7563503706022,8.92356415151605));
#10253=CARTESIAN_POINT('Ctrl Pts',(1.49961339720195,-12.7530891067545,9.1116890996567));
#10254=CARTESIAN_POINT('Ctrl Pts',(1.46164584377514,-12.7542036356865,9.31226849459714));
#10255=CARTESIAN_POINT('Ctrl Pts',(1.30822298061652,-12.7643815870671,9.68105805060626));
#10256=CARTESIAN_POINT('Ctrl Pts',(1.19277418140575,-12.7732022326273,9.8492775803417));
#10257=CARTESIAN_POINT('Ctrl Pts',(0.92667197373005,-12.7906121431377,10.114928217594));
#10258=CARTESIAN_POINT('Ctrl Pts',(0.758190528251416,-12.8003284816585,
10.2301098837158));
#10259=CARTESIAN_POINT('Ctrl Pts',(0.388988082274337,-12.8141939984886,
10.382902535549));
#10260=CARTESIAN_POINT('Ctrl Pts',(0.188255416016175,-12.8181093831741,
10.4205064589513));
#10261=CARTESIAN_POINT('Ctrl Pts',(-3.46944695195361E-16,-12.8181093831741,
10.4205064589513));
#10262=CARTESIAN_POINT('Origin',(0.,18.,8.9205064589513));
#10263=CARTESIAN_POINT('',(3.48148271110767E-13,12.8704745779592,7.42050645894779));
#10264=CARTESIAN_POINT('',(-5.11233613721112E-18,12.8181093831741,10.4205064589513));
#10265=CARTESIAN_POINT('Ctrl Pts',(-5.20417042793042E-16,12.8704745779587,
7.4205064589513));
#10266=CARTESIAN_POINT('Ctrl Pts',(-0.188854595603414,12.8704745779587,
7.4205064589513));
#10267=CARTESIAN_POINT('Ctrl Pts',(-0.390125974594806,12.8652326714021,
7.45834976030836));
#10268=CARTESIAN_POINT('Ctrl Pts',(-0.760025360862947,12.8460029733389,
7.61189577191482));
#10269=CARTESIAN_POINT('Ctrl Pts',(-0.9286705761767,12.8322493038568,7.72758625806842));
#10270=CARTESIAN_POINT('Ctrl Pts',(-1.19484729740032,12.8055313315293,7.9943061245009));
#10271=CARTESIAN_POINT('Ctrl Pts',(-1.31017366956046,12.7908167965405,8.16318338701933));
#10272=CARTESIAN_POINT('Ctrl Pts',(-1.46294688463921,12.7677413612085,8.53336354542309));
#10273=CARTESIAN_POINT('Ctrl Pts',(-1.50038190415455,12.7596246829664,8.73468650392867));
#10274=CARTESIAN_POINT('Ctrl Pts',(-1.49961339720195,12.7530891067545,9.1116890996567));
#10275=CARTESIAN_POINT('Ctrl Pts',(-1.46164584377514,12.7542036356865,9.31226849459714));
#10276=CARTESIAN_POINT('Ctrl Pts',(-1.30822298061652,12.7643815870671,9.68105805060626));
#10277=CARTESIAN_POINT('Ctrl Pts',(-1.19277418140575,12.7732022326273,9.8492775803417));
#10278=CARTESIAN_POINT('Ctrl Pts',(-0.92667197373005,12.7906121431377,10.114928217594));
#10279=CARTESIAN_POINT('Ctrl Pts',(-0.758190528251416,12.8003284816585,
10.2301098837158));
#10280=CARTESIAN_POINT('Ctrl Pts',(-0.388988082274336,12.8141939984886,
10.382902535549));
#10281=CARTESIAN_POINT('Ctrl Pts',(-0.188255416016174,12.8181093831741,
10.4205064589513));
#10282=CARTESIAN_POINT('Ctrl Pts',(1.73472347597681E-16,12.8181093831741,
10.4205064589513));
#10283=CARTESIAN_POINT('',(-1.83697019872103E-16,7.5,10.4205064589513));
#10284=CARTESIAN_POINT('',(-1.83697019872103E-16,18.,10.4205064589513));
#10285=CARTESIAN_POINT('Origin',(0.,7.5,8.9205064589513));
#10286=CARTESIAN_POINT('Ctrl Pts',(2.42861286636753E-16,12.8181093831741,
10.4205064589513));
#10287=CARTESIAN_POINT('Ctrl Pts',(0.188255416016175,12.8181093831741,10.4205064589513));
#10288=CARTESIAN_POINT('Ctrl Pts',(0.388988082274337,12.8141939984886,10.382902535549));
#10289=CARTESIAN_POINT('Ctrl Pts',(0.758190528251416,12.8003284816585,10.2301098837158));
#10290=CARTESIAN_POINT('Ctrl Pts',(0.92667197373005,12.7906121431377,10.114928217594));
#10291=CARTESIAN_POINT('Ctrl Pts',(1.19277418140575,12.7732022326273,9.8492775803417));
#10292=CARTESIAN_POINT('Ctrl Pts',(1.30822298061652,12.7643815870671,9.68105805060626));
#10293=CARTESIAN_POINT('Ctrl Pts',(1.46164584377514,12.7542036356865,9.31226849459714));
#10294=CARTESIAN_POINT('Ctrl Pts',(1.49961339720195,12.7530891067545,9.1116890996567));
#10295=CARTESIAN_POINT('Ctrl Pts',(1.49999688350216,12.7563503706022,8.92356415151605));
#10296=CARTESIAN_POINT('Ctrl Pts',(1.50038190415455,12.7596246829664,8.73468650392867));
#10297=CARTESIAN_POINT('Ctrl Pts',(1.46294688463921,12.7677413612085,8.53336354542309));
#10298=CARTESIAN_POINT('Ctrl Pts',(1.31017366956046,12.7908167965405,8.16318338701933));
#10299=CARTESIAN_POINT('Ctrl Pts',(1.19484729740032,12.8055313315293,7.9943061245009));
#10300=CARTESIAN_POINT('Ctrl Pts',(0.9286705761767,12.8322493038568,7.72758625806842));
#10301=CARTESIAN_POINT('Ctrl Pts',(0.760025360862947,12.8460029733389,7.61189577191482));
#10302=CARTESIAN_POINT('Ctrl Pts',(0.390125974594805,12.8652326714021,7.45834976030836));
#10303=CARTESIAN_POINT('Ctrl Pts',(0.188854595603413,12.8704745779587,7.4205064589513));
#10304=CARTESIAN_POINT('Ctrl Pts',(-3.12250225675825E-16,12.8704745779587,
7.4205064589513));
#10305=CARTESIAN_POINT('Origin',(0.,0.,0.));
#10306=CARTESIAN_POINT('',(10.3188329323468,7.5,13.9500588701352));
#10307=CARTESIAN_POINT('',(10.3188329323468,-7.5,13.9500588701352));
#10308=CARTESIAN_POINT('Origin',(0.,-3.20084840464449E-15,13.9500588701352));
#10309=CARTESIAN_POINT('',(10.5234605864397,7.5,4.43505886189467));
#10310=CARTESIAN_POINT('Ctrl Pts',(10.5234605864397,7.5,4.43505886189467));
#10311=CARTESIAN_POINT('Ctrl Pts',(10.4554775566161,7.5,7.60673038759669));
#10312=CARTESIAN_POINT('Ctrl Pts',(10.3872728229393,7.5,10.7783971699111));
#10313=CARTESIAN_POINT('Ctrl Pts',(10.3188329323468,7.5,13.9500588701352));
#10314=CARTESIAN_POINT('',(-12.2171188071335,4.42012220175077,0.45080521673159));
#10315=CARTESIAN_POINT('Ctrl Pts',(-12.2171188071335,4.42012220175077,0.45080521673159));
#10316=CARTESIAN_POINT('Ctrl Pts',(-12.149193478595,4.60591899525001,0.488759771825113));
#10317=CARTESIAN_POINT('Ctrl Pts',(-12.0770449733107,4.78999316985353,0.528777321711783));
#10318=CARTESIAN_POINT('Ctrl Pts',(-11.3399329531583,6.55066928002488,0.933845289815028));
#10319=CARTESIAN_POINT('Ctrl Pts',(-10.3575640140156,7.97284514437303,1.44149284263778));
#10320=CARTESIAN_POINT('Ctrl Pts',(-8.09951890179413,10.2431792877324,2.43522522106934));
#10321=CARTESIAN_POINT('Ctrl Pts',(-6.65236232722211,11.2433607265677,2.99343799717399));
#10322=CARTESIAN_POINT('Ctrl Pts',(-3.44419640635119,12.5847950346659,3.93990450984751));
#10323=CARTESIAN_POINT('Ctrl Pts',(-1.68108758943671,12.9245387443403,4.32317244135388));
#10324=CARTESIAN_POINT('Ctrl Pts',(0.803506534154167,12.9184636999382,4.67121150205686));
#10325=CARTESIAN_POINT('Ctrl Pts',(1.63698452641698,12.8407190060581,4.75873226104488));
#10326=CARTESIAN_POINT('Ctrl Pts',(3.29840062387174,12.515315106766,4.87233692567569));
#10327=CARTESIAN_POINT('Ctrl Pts',(4.12633991403241,12.2676894643164,4.89849962173473));
#10328=CARTESIAN_POINT('Ctrl Pts',(6.51022783913382,11.2852931824372,4.89403054082346));
#10329=CARTESIAN_POINT('Ctrl Pts',(7.96408954980376,10.2968570319164,4.77790964454782));
#10330=CARTESIAN_POINT('Ctrl Pts',(9.61578027154998,8.65854700523749,4.57553905407656));
#10331=CARTESIAN_POINT('Ctrl Pts',(10.0927434332412,8.10222543194356,4.50574481122557));
#10332=CARTESIAN_POINT('Ctrl Pts',(10.5234605864397,7.5,4.43505886189466));
#10333=CARTESIAN_POINT('',(-12.1056850526147,4.4201232096987,6.45080295373131));
#10334=CARTESIAN_POINT('Ctrl Pts',(-12.2171206478751,4.4201232096987,0.450804188182521));
#10335=CARTESIAN_POINT('Ctrl Pts',(-12.1982666930902,4.4201232096987,1.46639559259794));
#10336=CARTESIAN_POINT('Ctrl Pts',(-12.1794098522964,4.4201232096987,2.48198817833168));
#10337=CARTESIAN_POINT('Ctrl Pts',(-12.1605478920539,4.4201232096987,3.49758066897254));
#10338=CARTESIAN_POINT('Ctrl Pts',(-12.1422651106841,4.4201232096987,4.48198818698683));
#10339=CARTESIAN_POINT('Ctrl Pts',(-12.1239775194361,4.4201232096987,5.46639561565845));
#10340=CARTESIAN_POINT('Ctrl Pts',(-12.1056850526147,4.4201232096987,6.45080295373131));
#10341=CARTESIAN_POINT('',(-12.8874008156035,1.57825141581578E-15,6.45080295373131));
#10342=CARTESIAN_POINT('Origin',(0.,0.,6.45080295373131));
#10343=CARTESIAN_POINT('',(-12.4283466236009,9.69183562681548E-16,32.75));
#10344=CARTESIAN_POINT('',(-13.,1.59204083889156E-15,0.));
#10345=CARTESIAN_POINT('',(12.4283599700267,-2.15362009418406E-15,32.7492353837737));
#10346=CARTESIAN_POINT('Ctrl Pts',(-12.4283466236009,6.93889390390723E-16,
32.75));
#10347=CARTESIAN_POINT('Ctrl Pts',(-12.4283466236009,0.794308918128955,
32.75));
#10348=CARTESIAN_POINT('Ctrl Pts',(-12.3502527632816,1.61021372884421,32.7930538414047));
#10349=CARTESIAN_POINT('Ctrl Pts',(-12.0274177529636,3.22310913323241,32.9643815831464));
#10350=CARTESIAN_POINT('Ctrl Pts',(-11.7828051502509,4.0201542931032,33.0923838793489));
#10351=CARTESIAN_POINT('Ctrl Pts',(-10.8223388252417,6.3016876936436,33.5641120509972));
#10352=CARTESIAN_POINT('Ctrl Pts',(-9.86802331505246,7.67569650721005,33.9952885548655));
#10353=CARTESIAN_POINT('Ctrl Pts',(-7.68673433352581,9.84141368018456,34.7773406223861));
#10354=CARTESIAN_POINT('Ctrl Pts',(-6.30675051410171,10.7871492962387,35.1838249513449));
#10355=CARTESIAN_POINT('Ctrl Pts',(-4.01853645200771,11.7370350358201,35.6118527441021));
#10356=CARTESIAN_POINT('Ctrl Pts',(-3.21987048035003,11.9784899796951,35.7251137378412));
#10357=CARTESIAN_POINT('Ctrl Pts',(-1.60639827951172,12.2965977499602,35.8754701561768));
#10358=CARTESIAN_POINT('Ctrl Pts',(-0.791562918351071,12.3731454095824,
35.9124754330905));
#10359=CARTESIAN_POINT('Ctrl Pts',(0.791571803892222,12.3731461491244,35.9124330647567));
#10360=CARTESIAN_POINT('Ctrl Pts',(1.60641400117091,12.296597562387,35.875383360731));
#10361=CARTESIAN_POINT('Ctrl Pts',(3.21989600364048,11.9784866527797,35.7249372434734));
#10362=CARTESIAN_POINT('Ctrl Pts',(4.01856495072364,11.7370295233017,35.6116309738994));
#10363=CARTESIAN_POINT('Ctrl Pts',(6.30678393558675,10.7871375666671,35.1834705050684));
#10364=CARTESIAN_POINT('Ctrl Pts',(7.68676566759693,9.84139890551597,34.7769017525103));
#10365=CARTESIAN_POINT('Ctrl Pts',(9.8680427591823,7.67568550857489,33.9947109969587));
#10366=CARTESIAN_POINT('Ctrl Pts',(10.8223529970034,6.30168425346591,33.5634693670658));
#10367=CARTESIAN_POINT('Ctrl Pts',(11.7828170674242,4.02015736730738,33.0916705623065));
#10368=CARTESIAN_POINT('Ctrl Pts',(12.0274298028565,3.22311347643651,32.9636492417211));
#10369=CARTESIAN_POINT('Ctrl Pts',(12.3502655341755,1.61021795970926,32.7922958208113));
#10370=CARTESIAN_POINT('Ctrl Pts',(12.4283599700267,0.794311754446631,32.7492353837737));
#10371=CARTESIAN_POINT('Ctrl Pts',(12.4283599700267,1.38777878078145E-16,
32.7492353837737));
#10372=CARTESIAN_POINT('Ctrl Pts',(12.4283599700267,-2.77555756156289E-16,
32.7492353837737));
#10373=CARTESIAN_POINT('Ctrl Pts',(12.4283599700267,-0.794311754446632,
32.7492353837737));
#10374=CARTESIAN_POINT('Ctrl Pts',(12.3502655341755,-1.61021795970926,32.7922958208113));
#10375=CARTESIAN_POINT('Ctrl Pts',(12.0274298028565,-3.22311347643651,32.9636492417211));
#10376=CARTESIAN_POINT('Ctrl Pts',(11.7828170674242,-4.02015736730738,33.0916705623065));
#10377=CARTESIAN_POINT('Ctrl Pts',(10.8223529970034,-6.30168425346592,33.5634693670658));
#10378=CARTESIAN_POINT('Ctrl Pts',(9.8680427591823,-7.6756855085749,33.9947109969587));
#10379=CARTESIAN_POINT('Ctrl Pts',(7.68676566759692,-9.84139890551598,34.7769017525103));
#10380=CARTESIAN_POINT('Ctrl Pts',(6.30678393558675,-10.7871375666671,35.1834705050684));
#10381=CARTESIAN_POINT('Ctrl Pts',(4.01856495072364,-11.7370295233017,35.6116309738994));
#10382=CARTESIAN_POINT('Ctrl Pts',(3.21989600364047,-11.9784866527797,35.7249372434734));
#10383=CARTESIAN_POINT('Ctrl Pts',(1.60641400117091,-12.296597562387,35.875383360731));
#10384=CARTESIAN_POINT('Ctrl Pts',(0.791571803892224,-12.3731461491244,
35.9124330647567));
#10385=CARTESIAN_POINT('Ctrl Pts',(-0.791562918351067,-12.3731454095824,
35.9124754330905));
#10386=CARTESIAN_POINT('Ctrl Pts',(-1.60639827951171,-12.2965977499602,
35.8754701561768));
#10387=CARTESIAN_POINT('Ctrl Pts',(-3.21987048035002,-11.9784899796951,
35.7251137378412));
#10388=CARTESIAN_POINT('Ctrl Pts',(-4.0185364520077,-11.7370350358201,35.6118527441021));
#10389=CARTESIAN_POINT('Ctrl Pts',(-6.30675051410171,-10.7871492962387,
35.1838249513449));
#10390=CARTESIAN_POINT('Ctrl Pts',(-7.68673433352581,-9.84141368018457,
34.7773406223861));
#10391=CARTESIAN_POINT('Ctrl Pts',(-9.86802331505246,-7.67569650721005,
33.9952885548655));
#10392=CARTESIAN_POINT('Ctrl Pts',(-10.8223388252417,-6.3016876936436,33.5641120509972));
#10393=CARTESIAN_POINT('Ctrl Pts',(-11.7828051502509,-4.0201542931032,33.0923838793489));
#10394=CARTESIAN_POINT('Ctrl Pts',(-12.0274177529636,-3.22310913323241,
32.9643815831464));
#10395=CARTESIAN_POINT('Ctrl Pts',(-12.3502527632816,-1.61021372884421,
32.7930538414047));
#10396=CARTESIAN_POINT('Ctrl Pts',(-12.4283466236009,-0.794308918128954,
32.75));
#10397=CARTESIAN_POINT('Ctrl Pts',(-12.4283466236009,0.,32.75));
#10398=CARTESIAN_POINT('',(-12.1056850526147,-4.4201232096987,6.45080295373131));
#10399=CARTESIAN_POINT('Origin',(0.,0.,6.45080295373131));
#10400=CARTESIAN_POINT('',(-12.2171192862399,-4.4201226050411,0.450804099959431));
#10401=CARTESIAN_POINT('Ctrl Pts',(-12.1056850526147,-4.4201232096987,6.45080295373131));
#10402=CARTESIAN_POINT('Ctrl Pts',(-12.1239775194361,-4.4201232096987,5.46639561565844));
#10403=CARTESIAN_POINT('Ctrl Pts',(-12.1422651106866,-4.4201232096987,4.48198818697493));
#10404=CARTESIAN_POINT('Ctrl Pts',(-12.1605478920564,-4.4201232096987,3.49758066896046));
#10405=CARTESIAN_POINT('Ctrl Pts',(-12.179409852299,-4.4201232096987,2.48198817831942));
#10406=CARTESIAN_POINT('Ctrl Pts',(-12.1982666930902,-4.4201232096987,1.46639559259794));
#10407=CARTESIAN_POINT('Ctrl Pts',(-12.2171206478751,-4.4201232096987,0.45080418818252));
#10408=CARTESIAN_POINT('',(10.5234605864397,-7.5,4.43505886189467));
#10409=CARTESIAN_POINT('Ctrl Pts',(10.5234605864397,-7.50000000000001,4.43505886189466));
#10410=CARTESIAN_POINT('Ctrl Pts',(10.0927434332412,-8.10222543194357,4.50574481122557));
#10411=CARTESIAN_POINT('Ctrl Pts',(9.61578027154998,-8.6585470052375,4.57553905407656));
#10412=CARTESIAN_POINT('Ctrl Pts',(7.96408954980375,-10.2968570319164,4.77790964454782));
#10413=CARTESIAN_POINT('Ctrl Pts',(6.51022783913381,-11.2852931824372,4.89403054082346));
#10414=CARTESIAN_POINT('Ctrl Pts',(4.1263399140324,-12.2676894643164,4.89849962173473));
#10415=CARTESIAN_POINT('Ctrl Pts',(3.29840062387173,-12.515315106766,4.87233692567569));
#10416=CARTESIAN_POINT('Ctrl Pts',(1.63698452641698,-12.8407190060581,4.75873226104488));
#10417=CARTESIAN_POINT('Ctrl Pts',(0.803506534154166,-12.9184636999382,
4.67121150205686));
#10418=CARTESIAN_POINT('Ctrl Pts',(-1.68108758943671,-12.9245387443403,
4.32317244135388));
#10419=CARTESIAN_POINT('Ctrl Pts',(-3.44419640635119,-12.5847950346659,
3.93990450984751));
#10420=CARTESIAN_POINT('Ctrl Pts',(-6.6523623272221,-11.2433607265677,2.99343799717399));
#10421=CARTESIAN_POINT('Ctrl Pts',(-8.09951890179412,-10.2431792877324,
2.43522522106934));
#10422=CARTESIAN_POINT('Ctrl Pts',(-10.3575640140156,-7.97284514437303,
1.44149284263779));
#10423=CARTESIAN_POINT('Ctrl Pts',(-11.3399329531583,-6.55066928002488,
0.933845289815027));
#10424=CARTESIAN_POINT('Ctrl Pts',(-12.0770449733107,-4.78999316985353,
0.528777321711782));
#10425=CARTESIAN_POINT('Ctrl Pts',(-12.149193478595,-4.60591899525002,0.488759771825114));
#10426=CARTESIAN_POINT('Ctrl Pts',(-12.2171188071335,-4.42012220175077,
0.450805216731591));
#10427=CARTESIAN_POINT('Ctrl Pts',(10.3188329323468,-7.5,13.9500588701352));
#10428=CARTESIAN_POINT('Ctrl Pts',(10.3872728229393,-7.5,10.7783971699111));
#10429=CARTESIAN_POINT('Ctrl Pts',(10.4554775566161,-7.5,7.60673038759669));
#10430=CARTESIAN_POINT('Ctrl Pts',(10.5234605864397,-7.5,4.43505886189467));
#10431=CARTESIAN_POINT('Origin',(-12.4644660428009,2.5,-2.91315807694762));
#10432=CARTESIAN_POINT('',(-15.1213202922933,-2.5,-0.256303827455243));
#10433=CARTESIAN_POINT('',(-12.4644660428009,-2.5,-2.91315807694762));
#10434=CARTESIAN_POINT('',(-15.1213202922933,2.5,-0.256303827455242));
#10435=CARTESIAN_POINT('Origin',(-19.5355338546664,-2.5,-9.9842258888131));
#10436=CARTESIAN_POINT('',(-13.7071067299202,-2.5,-0.256303827455243));
#10437=CARTESIAN_POINT('',(-17.9497474170395,-2.5,-4.49894451457453));
#10438=CARTESIAN_POINT('Origin',(-14.4142135111068,-2.5,0.450802953731305));
#10439=CARTESIAN_POINT('Origin',(-19.5355338546664,2.5,-9.9842258888131));
#10440=CARTESIAN_POINT('',(-15.1213202922933,2.5,-0.256303827455243));
#10441=CARTESIAN_POINT('',(-12.4644660428009,2.5,-2.91315807694762));
#10442=CARTESIAN_POINT('',(-13.7071067299202,2.5,-0.256303827455243));
#10443=CARTESIAN_POINT('',(-17.9497474170395,2.5,-4.49894451457453));
#10444=CARTESIAN_POINT('Origin',(-14.4142135111068,2.5,0.450802953731305));
#10445=CARTESIAN_POINT('Origin',(-11.224345965807,0.,-11.224345965807));
#10446=CARTESIAN_POINT('',(-18.656854198226,-4.4201232096987,-3.79183773338798));
#10447=CARTESIAN_POINT('',(-20.242640635853,-4.4201232096987,-2.20605129576108));
#10448=CARTESIAN_POINT('',(-17.9497474170395,-4.4201232096987,-4.49894451457453));
#10449=CARTESIAN_POINT('',(-20.242640635853,-2.5,-2.20605129576108));
#10450=CARTESIAN_POINT('',(-20.242640635853,-2.5,-2.20605129576108));
#10451=CARTESIAN_POINT('',(-18.656854198226,-2.5,-3.79183773338798));
#10452=CARTESIAN_POINT('',(-11.224345965807,-2.5,-11.224345965807));
#10453=CARTESIAN_POINT('',(-18.656854198226,-4.4201232096987,-3.79183773338798));
#10454=CARTESIAN_POINT('Origin',(0.,0.,0.));
#10455=CARTESIAN_POINT('Origin',(0.,0.,0.450802953731306));
#10456=CARTESIAN_POINT('Ctrl Pts',(-12.2171188071335,-4.42012220175077,
0.450805216731591));
#10457=CARTESIAN_POINT('Ctrl Pts',(-12.4437244891765,-3.80028553672204,
0.324185029112939));
#10458=CARTESIAN_POINT('Ctrl Pts',(-12.6230045022273,-3.16110024476212,
0.220809942356288));
#10459=CARTESIAN_POINT('Ctrl Pts',(-12.9188641006425,-1.67701333832259,
0.0485983978862804));
#10460=CARTESIAN_POINT('Ctrl Pts',(-13.,-0.827603999929081,-8.71233909165408E-15));
#10461=CARTESIAN_POINT('Ctrl Pts',(-13.,0.827603999929072,-9.05122930234842E-15));
#10462=CARTESIAN_POINT('Ctrl Pts',(-12.9188641006425,1.67701333832258,0.0485983978862817));
#10463=CARTESIAN_POINT('Ctrl Pts',(-12.6230045022273,3.16110024476212,0.22080994235629));
#10464=CARTESIAN_POINT('Ctrl Pts',(-12.4437244891765,3.80028553672204,0.324185029112938));
#10465=CARTESIAN_POINT('Ctrl Pts',(-12.2171188071335,4.42012220175077,0.45080521673159));
#10466=CARTESIAN_POINT('Origin',(4.85535470457189,36.,-30.1029285680633));
#10467=CARTESIAN_POINT('',(-8.,-7.5,2.45071724035024));
#10468=CARTESIAN_POINT('',(-8.,7.5,2.45071724035023));
#10469=CARTESIAN_POINT('',(-8.,36.,2.45071724035024));
#10470=CARTESIAN_POINT('Origin',(4.85535470457189,-7.5,-30.1029285680633));
#10471=CARTESIAN_POINT('Origin',(4.85535470457189,7.5,-30.1029285680633));
#10472=CARTESIAN_POINT('Origin',(-0.000695819921353427,36.,9.91245425835333));
#10473=CARTESIAN_POINT('',(7.44355606790684,-4.4201232096987,34.8239599099708));
#10474=CARTESIAN_POINT('',(7.44355606790684,4.4201232096987,34.8239599099708));
#10475=CARTESIAN_POINT('',(7.44355606790684,36.,34.8239599099708));
#10476=CARTESIAN_POINT('',(-7.44355606790684,-4.4201232096987,34.8243757283837));
#10477=CARTESIAN_POINT('Origin',(-0.000695819921353427,-4.4201232096987,
9.91245425835333));
#10478=CARTESIAN_POINT('',(-7.44355606790684,4.4201232096987,34.8243757283837));
#10479=CARTESIAN_POINT('',(-7.44355606790684,36.,34.8243757283837));
#10480=CARTESIAN_POINT('Origin',(-0.000695819921353427,4.4201232096987,
9.91245425835333));
#10481=CARTESIAN_POINT('Origin',(16.,7.5,13.9500588701352));
#10482=CARTESIAN_POINT('',(-8.,-7.5,13.9500588701352));
#10483=CARTESIAN_POINT('',(16.,-7.5,13.9500588701352));
#10484=CARTESIAN_POINT('',(-8.,7.5,13.9500588701352));
#10485=CARTESIAN_POINT('',(-8.,7.5,13.9500588701352));
#10486=CARTESIAN_POINT('',(16.,7.5,13.9500588701352));
#10487=CARTESIAN_POINT('Origin',(16.,-7.5,-13.9500588701352));
#10488=CARTESIAN_POINT('',(-8.,-7.5,-13.9500588701352));
#10489=CARTESIAN_POINT('Origin',(16.,7.5,-13.9500588701352));
#10490=CARTESIAN_POINT('',(-8.,7.5,-13.9500588701352));
#10491=CARTESIAN_POINT('Origin',(-8.,0.,0.));
#10492=CARTESIAN_POINT('Origin',(13.2559086557882,-4.4201232096987,0.450802953731306));
#10493=CARTESIAN_POINT('',(-12.9999999487337,-4.4201232096987,0.450802953731307));
#10494=CARTESIAN_POINT('',(13.2559086557882,-4.4201232096987,0.450802953731306));
#10495=CARTESIAN_POINT('',(-12.9999999487337,4.4201232096987,0.450802953731308));
#10496=CARTESIAN_POINT('',(-12.9999999487337,-4.4201232096987,0.450802953731306));
#10497=CARTESIAN_POINT('',(13.2559086557882,4.4201232096987,0.450802953731306));
#10498=CARTESIAN_POINT('Origin',(13.2559086557882,4.4201232096987,6.45080295373131));
#10499=CARTESIAN_POINT('',(-20.242640635853,4.4201232096987,-2.20605129576108));
#10500=CARTESIAN_POINT('',(-18.656854198226,4.4201232096987,-3.79183773338798));
#10501=CARTESIAN_POINT('',(-20.9497474170395,4.4201232096987,-1.49894451457453));
#10502=CARTESIAN_POINT('',(-20.242640635853,4.4201232096987,-0.79183773338798));
#10503=CARTESIAN_POINT('Origin',(-19.5355338546664,4.4201232096987,-1.49894451457453));
#10504=CARTESIAN_POINT('',(-12.9999999487337,4.4201232096987,6.45080295373131));
#10505=CARTESIAN_POINT('',(-20.9497474170395,4.4201232096987,-1.49894451457453));
#10506=CARTESIAN_POINT('',(13.2559086557882,4.4201232096987,6.45080295373131));
#10507=CARTESIAN_POINT('',(-17.2426406358529,4.4201232096987,-3.79183773338798));
#10508=CARTESIAN_POINT('',(-17.9497474170395,4.4201232096987,-4.49894451457453));
#10509=CARTESIAN_POINT('Origin',(-17.9497474170395,4.4201232096987,-3.08473095220143));
#10510=CARTESIAN_POINT('Origin',(13.2559086557882,-4.4201232096987,6.45080295373131));
#10511=CARTESIAN_POINT('',(-12.9999999487337,-4.4201232096987,6.45080295373131));
#10512=CARTESIAN_POINT('',(-12.9999999487337,-4.4201232096987,6.45080295373131));
#10513=CARTESIAN_POINT('',(13.2559086557882,-4.4201232096987,6.45080295373131));
#10514=CARTESIAN_POINT('Origin',(13.2559086557882,-4.4201232096987,6.45080295373131));
#10515=CARTESIAN_POINT('',(-20.242640635853,-4.4201232096987,-0.79183773338798));
#10516=CARTESIAN_POINT('',(-20.9497474170395,-4.4201232096987,-1.49894451457453));
#10517=CARTESIAN_POINT('Origin',(-19.5355338546664,-4.4201232096987,-1.49894451457453));
#10518=CARTESIAN_POINT('',(-17.2426406358529,-4.4201232096987,-3.79183773338798));
#10519=CARTESIAN_POINT('Origin',(-17.9497474170395,-4.4201232096987,-3.08473095220143));
#10520=CARTESIAN_POINT('',(-17.9497474170395,-4.4201232096987,-4.49894451457453));
#10521=CARTESIAN_POINT('Origin',(-17.9497474170395,4.4201232096987,-4.49894451457453));
#10522=CARTESIAN_POINT('',(-17.2426406358529,2.5,-3.79183773338798));
#10523=CARTESIAN_POINT('',(-17.9497474170395,2.5,-4.49894451457453));
#10524=CARTESIAN_POINT('',(-17.2426406358529,4.4201232096987,-3.79183773338798));
#10525=CARTESIAN_POINT('',(-17.2426406358529,-2.5,-3.79183773338798));
#10526=CARTESIAN_POINT('',(-17.2426406358529,-2.5,-3.79183773338798));
#10527=CARTESIAN_POINT('',(-17.9497474170395,-2.5,-4.49894451457453));
#10528=CARTESIAN_POINT('',(-13.7071067299202,4.4201232096987,-0.256303827455243));
#10529=CARTESIAN_POINT('Origin',(-20.9497474170395,-4.4201232096987,-1.49894451457453));
#10530=CARTESIAN_POINT('',(-20.242640635853,2.5,-0.791837733387981));
#10531=CARTESIAN_POINT('',(-24.4852813229722,2.5,-5.03447842050726));
#10532=CARTESIAN_POINT('',(-20.242640635853,-2.5,-0.791837733387981));
#10533=CARTESIAN_POINT('',(-24.4852813229722,-2.5,-5.03447842050726));
#10534=CARTESIAN_POINT('',(-20.242640635853,-4.4201232096987,-0.79183773338798));
#10535=CARTESIAN_POINT('',(-20.242640635853,2.5,-0.79183773338798));
#10536=CARTESIAN_POINT('Origin',(-11.224345965807,0.,-11.224345965807));
#10537=CARTESIAN_POINT('',(-20.242640635853,2.5,-2.20605129576108));
#10538=CARTESIAN_POINT('',(-18.656854198226,2.5,-3.79183773338798));
#10539=CARTESIAN_POINT('',(-11.224345965807,2.5,-11.224345965807));
#10540=CARTESIAN_POINT('',(-20.242640635853,4.4201232096987,-2.20605129576108));
#10541=CARTESIAN_POINT('',(-18.656854198226,2.5,-3.79183773338798));
#10542=CARTESIAN_POINT('Origin',(-12.4644660428009,2.5,-2.91315807694762));
#10543=CARTESIAN_POINT('',(-15.1213202922933,2.5,-0.256303827455242));
#10544=CARTESIAN_POINT('Origin',(-19.5355338546664,-2.5,-9.9842258888131));
#10545=CARTESIAN_POINT('Origin',(-17.9497474170395,-2.5,-3.08473095220143));
#10546=CARTESIAN_POINT('Origin',(-19.5355338546664,-2.5,-1.49894451457453));
#10547=CARTESIAN_POINT('Origin',(-19.5355338546664,2.5,-9.9842258888131));
#10548=CARTESIAN_POINT('Origin',(-19.5355338546664,2.5,-1.49894451457453));
#10549=CARTESIAN_POINT('Origin',(-17.9497474170395,2.5,-3.08473095220143));
#10550=CARTESIAN_POINT('Origin',(-18.0355338546664,-5.4201232096987,-1.58473095220143));
#10551=CARTESIAN_POINT('Origin',(-18.0355338546664,5.4198767903013,-1.58473095220143));
#10552=CARTESIAN_POINT('Origin',(-19.5355338546664,0.,-1.49894451457453));
#10553=CARTESIAN_POINT('Origin',(-19.5355338546664,0.,-1.49894451457453));
#10554=CARTESIAN_POINT('Origin',(-17.9497474170395,0.,-3.08473095220143));
#10555=CARTESIAN_POINT('Origin',(-17.9497474170395,0.,-3.08473095220143));
#10556=CARTESIAN_POINT('Origin',(-14.4142135111068,4.4201232096987,0.450802953731305));
#10557=CARTESIAN_POINT('Origin',(0.,0.,45.));
#10558=CARTESIAN_POINT('',(-4.44355606790684,-4.4201232096987,45.));
#10559=CARTESIAN_POINT('',(4.44355606790684,-4.4201232096987,45.));
#10560=CARTESIAN_POINT('',(7.44355606790684,-4.4201232096987,45.));
#10561=CARTESIAN_POINT('',(4.44355606790684,4.4201232096987,45.));
#10562=CARTESIAN_POINT('',(4.44355606790684,4.4201232096987,45.));
#10563=CARTESIAN_POINT('',(-4.44355606790684,4.4201232096987,45.));
#10564=CARTESIAN_POINT('',(7.44355606790684,4.4201232096987,45.));
#10565=CARTESIAN_POINT('',(-4.44355606790684,-4.4201232096987,45.));
#10566=CARTESIAN_POINT('Origin',(7.44355606790684,-4.4201232096987,-4.08573095220143));
#10567=CARTESIAN_POINT('',(7.44355606790684,-4.4201232096987,42.));
#10568=CARTESIAN_POINT('',(7.44355606790684,-4.4201232096987,-4.08573095220143));
#10569=CARTESIAN_POINT('Origin',(4.44355606790684,-4.4201232096987,42.));
#10570=CARTESIAN_POINT('',(-7.44355606790684,-4.4201232096987,42.));
#10571=CARTESIAN_POINT('Origin',(-4.44355606790684,-4.4201232096987,42.));
#10572=CARTESIAN_POINT('',(-7.44355606790684,-4.4201232096987,-4.08573095220143));
#10573=CARTESIAN_POINT('Origin',(7.44355606790684,4.4201232096987,-4.08573095220143));
#10574=CARTESIAN_POINT('',(7.44355606790684,4.4201232096987,42.));
#10575=CARTESIAN_POINT('',(7.44355606790684,4.4201232096987,-4.08573095220143));
#10576=CARTESIAN_POINT('',(7.44355606790684,-4.4201232096987,42.));
#10577=CARTESIAN_POINT('Origin',(7.44355606790684,4.4201232096987,-4.08573095220143));
#10578=CARTESIAN_POINT('Origin',(4.44355606790684,4.4201232096987,42.));
#10579=CARTESIAN_POINT('',(-7.44355606790684,4.4201232096987,42.));
#10580=CARTESIAN_POINT('',(-7.44355606790684,4.4201232096987,-4.08573095220143));
#10581=CARTESIAN_POINT('Origin',(-4.44355606790684,4.4201232096987,42.));
#10582=CARTESIAN_POINT('Origin',(-7.44355606790684,4.4201232096987,-4.08573095220143));
#10583=CARTESIAN_POINT('',(-7.44355606790684,4.4201232096987,42.));
#10584=CARTESIAN_POINT('Origin',(4.44355606790684,0.,42.));
#10585=CARTESIAN_POINT('Origin',(-4.44355606790684,0.,42.));
#13151=UNCERTAINTY_MEASURE_WITH_UNIT(LENGTH_MEASURE(0.01),#13200,
'DISTANCE_ACCURACY_VALUE',
'Maximum model space distance between geometric entities at asserted c
onnectivities');
#13173=UNCERTAINTY_MEASURE_WITH_UNIT(LENGTH_MEASURE(0.01),#13200,
'DISTANCE_ACCURACY_VALUE',
'Maximum model space distance between geometric entities at asserted c
onnectivities');
#13177=(
GEOMETRIC_REPRESENTATION_CONTEXT(3)
GLOBAL_UNCERTAINTY_ASSIGNED_CONTEXT((#13151))
GLOBAL_UNIT_ASSIGNED_CONTEXT((#13200,#13202,#13203))
REPRESENTATION_CONTEXT('','3D')
);
#13199=(
GEOMETRIC_REPRESENTATION_CONTEXT(3)
GLOBAL_UNCERTAINTY_ASSIGNED_CONTEXT((#13173))
GLOBAL_UNIT_ASSIGNED_CONTEXT((#13200,#13202,#13203))
REPRESENTATION_CONTEXT('','3D')
);
#13200=(
LENGTH_UNIT()
NAMED_UNIT(*)
SI_UNIT(.MILLI.,.METRE.)
);
#13202=(
NAMED_UNIT(*)
PLANE_ANGLE_UNIT()
SI_UNIT($,.RADIAN.)
);
#13203=(
NAMED_UNIT(*)
SI_UNIT($,.STERADIAN.)
SOLID_ANGLE_UNIT()
);
#13207=SHAPE_DEFINITION_REPRESENTATION(#13232,#13281);
#13232=PRODUCT_DEFINITION_SHAPE('',$,#13307);
#13281=SHAPE_REPRESENTATION('',(#7193),#13177);
#13303=PRODUCT_DEFINITION_CONTEXT('part definition',#13380,'design');
#13307=PRODUCT_DEFINITION('Finger Link 1','Finger Link 1',#13332,#13303);
#13332=PRODUCT_DEFINITION_FORMATION('',$,#13385);
#13380=APPLICATION_CONTEXT(
'Core Data for Automotive Mechanical Design Process');
#13381=PRODUCT_CONTEXT('part definition',#13380,'mechanical');
#13385=PRODUCT('Finger Link 1','Finger Link 1',$,(#13381));
#13409=PRESENTATION_STYLE_ASSIGNMENT((#13414));
#13414=SURFACE_STYLE_USAGE(.BOTH.,#13419);
#13419=SURFACE_SIDE_STYLE('',(#13424));
#13424=SURFACE_STYLE_FILL_AREA(#13429);
#13429=FILL_AREA_STYLE('Opaque(61,176,222)',(#13434));
#13434=FILL_AREA_STYLE_COLOUR('Opaque(61,176,222)',#13439);
#13439=COLOUR_RGB('Opaque(61,176,222)',0.23921568627451,0.690196078431373,
0.870588235294118);
ENDSEC;
END-ISO-10303-21;
